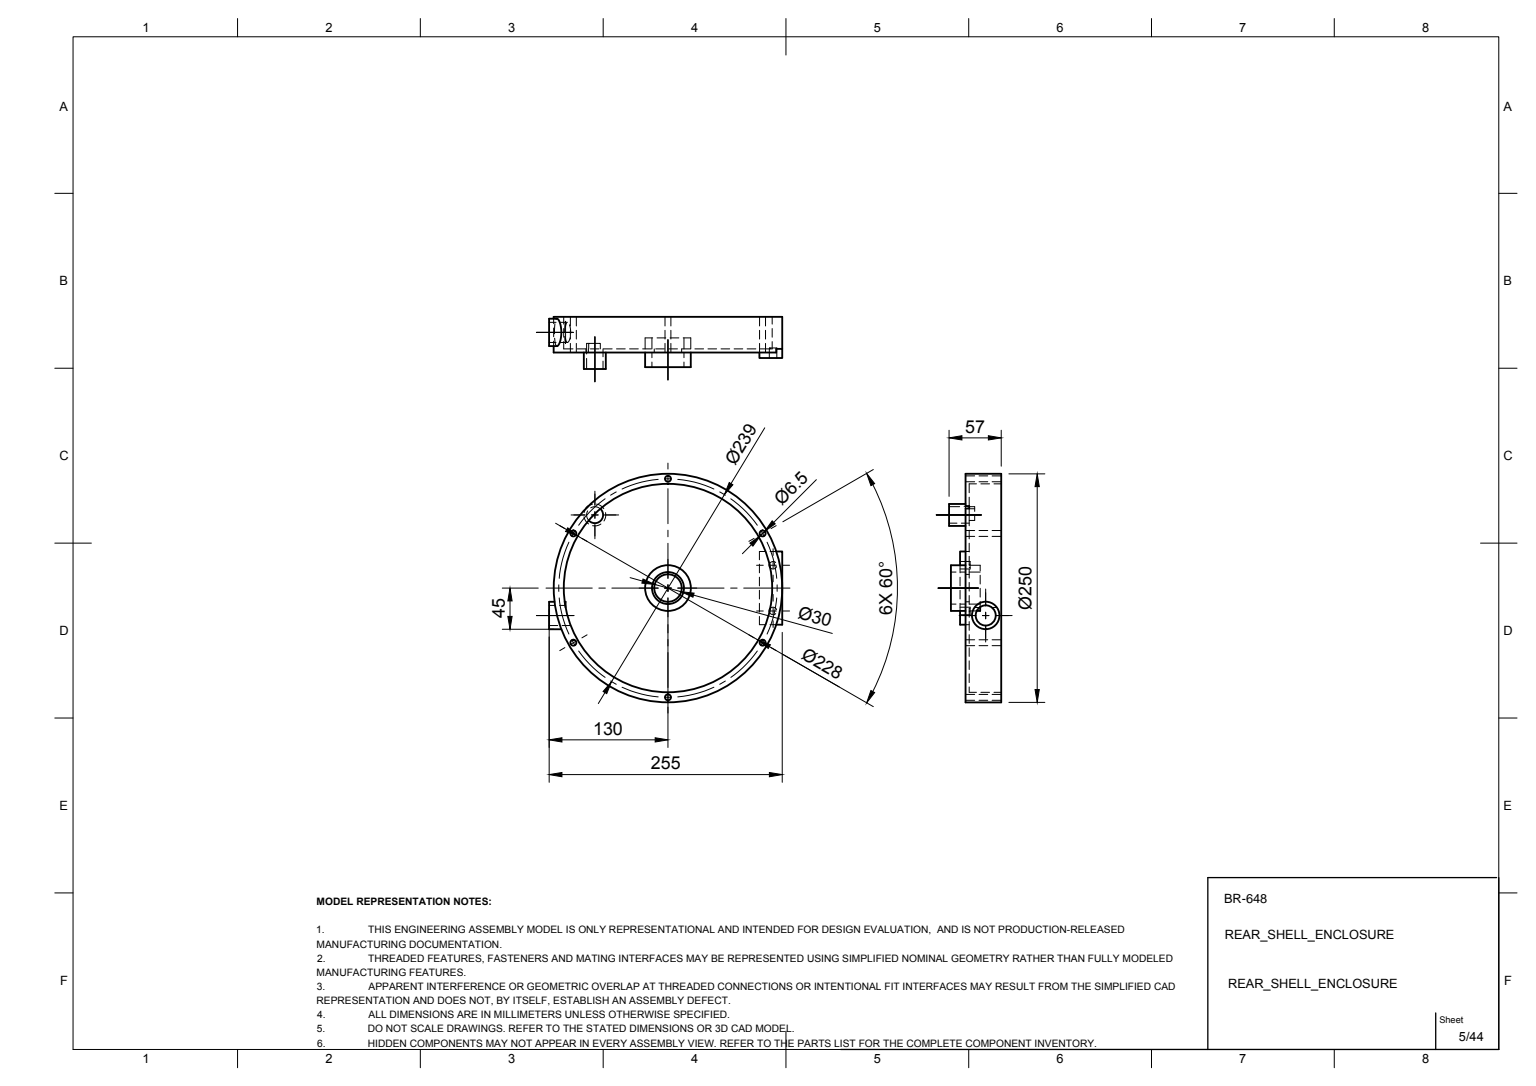
ISO-10303-21;
HEADER;
FILE_DESCRIPTION((''),'2;1');
FILE_NAME('REAR_SHELL_ENCLOSURE.step','2026-10-01T22:05:39-07:00',(''),(''),'','','');
FILE_SCHEMA (('AUTOMOTIVE_DESIGN { 1 0 10303 214 3 1 1 }'));
ENDSEC;
DATA;
#10=MECHANICAL_DESIGN_GEOMETRIC_PRESENTATION_REPRESENTATION('',(#605),#24628);
#521=SHAPE_REPRESENTATION_RELATIONSHIP('SRR','None',#24793,#563) ;
#563=ADVANCED_BREP_SHAPE_REPRESENTATION('',(#647),#24583) ;
#605=STYLED_ITEM('',(#25031),#647) ;
#647=MANIFOLD_SOLID_BREP('REAR_SHELL_ENCLOSURE',#13114) ;
#686=FACE_BOUND('',#3722,.T.) ;
#687=FACE_BOUND('',#3726,.T.) ;
#688=FACE_BOUND('',#3738,.T.) ;
#689=FACE_BOUND('',#3739,.T.) ;
#690=FACE_BOUND('',#3743,.T.) ;
#691=FACE_BOUND('',#3748,.T.) ;
#692=FACE_BOUND('',#3755,.T.) ;
#693=FACE_BOUND('',#3757,.T.) ;
#694=FACE_BOUND('',#3758,.T.) ;
#695=FACE_BOUND('',#3759,.T.) ;
#696=FACE_BOUND('',#3760,.T.) ;
#697=FACE_BOUND('',#3761,.T.) ;
#698=FACE_BOUND('',#3762,.T.) ;
#699=FACE_BOUND('',#3763,.T.) ;
#700=FACE_BOUND('',#3767,.T.) ;
#701=FACE_BOUND('',#3770,.T.) ;
#702=FACE_BOUND('',#3773,.T.) ;
#703=FACE_BOUND('',#3776,.T.) ;
#704=FACE_BOUND('',#3778,.T.) ;
#705=FACE_BOUND('',#3779,.T.) ;
#706=FACE_BOUND('',#3780,.T.) ;
#707=FACE_BOUND('',#3781,.T.) ;
#708=FACE_BOUND('',#3782,.T.) ;
#709=FACE_BOUND('',#3783,.T.) ;
#710=FACE_BOUND('',#3784,.T.) ;
#951=B_SPLINE_CURVE_WITH_KNOTS('',3,(#19746,#19747,#19748,#19749,#19750,
#19751,#19752,#19753,#19754,#19755,#19756,#19757,#19758,#19759,#19760,#19761),
 .UNSPECIFIED.,.F.,.F.,(4,2,2,2,2,2,2,4),(0.687250434098959,0.82687421960189,
1.25301704446935,1.67915986933681,2.11450443098489,2.54984899263297,2.96432241698031,
3.37879584132764),.UNSPECIFIED.) ;
#952=B_SPLINE_CURVE_WITH_KNOTS('',3,(#19763,#19764,#19765,#19766,#19767,
#19768,#19769,#19770,#19771,#19772,#19773,#19774,#19775,#19776,#19777,#19778),
 .UNSPECIFIED.,.F.,.F.,(4,2,2,2,2,2,2,4),(3.37879584132764,3.79326926567498,
4.20774269002231,4.6430872516704,5.07843181331848,5.50457463818594,5.9307174630534,
6.07034124855633),.UNSPECIFIED.) ;
#953=B_SPLINE_CURVE_WITH_KNOTS('',3,(#19782,#19783,#19784,#19785,#19786,
#19787,#19788,#19789,#19790,#19791,#19792,#19793,#19794,#19795,#19796,#19797,
#19798,#19799,#19800,#19801,#19802,#19803,#19804),.UNSPECIFIED.,.F.,.F.,
(4,2,2,2,2,3,2,2,2,2,4),(-1.37470917955979,-1.12781391794867,-0.8458604384615,
-0.563906958974332,-0.281953479487166,0.,0.281953479487167,0.563906958974333,
0.8458604384615,1.12781391794867,1.37470917955955),.UNSPECIFIED.) ;
#954=B_SPLINE_CURVE_WITH_KNOTS('',3,(#19913,#19914,#19915,#19916,#19917,
#19918,#19919,#19920,#19921,#19922,#19923,#19924,#19925,#19926,#19927,#19928,
#19929,#19930,#19931,#19932,#19933,#19934,#19935,#19936,#19937,#19938),
 .UNSPECIFIED.,.F.,.F.,(4,2,2,2,2,2,2,2,2,2,2,2,4),(0.,0.56410198036302,
0.84615297054453,1.12820396072604,1.41660602376442,1.7050080868028,1.99341014984119,
2.28181221287957,2.87260145541368,3.46339069794779,4.02908355018852,4.31192997630889,
4.59477640242925),.UNSPECIFIED.) ;
#955=B_SPLINE_CURVE_WITH_KNOTS('',3,(#19939,#19940,#19941,#19942,#19943,
#19944,#19945,#19946,#19947,#19948,#19949,#19950,#19951,#19952,#19953,#19954,
#19955,#19956,#19957,#19958,#19959,#19960,#19961,#19962,#19963,#19964),
 .UNSPECIFIED.,.F.,.F.,(4,2,2,2,2,2,2,2,2,2,2,2,4),(4.59477640242925,4.87762282854962,
5.16046925466999,5.72616210691072,6.31695134944483,6.90774059197894,7.19614265501732,
7.4845447180557,7.77294678109409,8.06134884413247,8.34339983431398,8.62545082449549,
9.18955280485851),.UNSPECIFIED.) ;
#1001=LINE('',#19715,#1837) ;
#1002=LINE('',#19717,#1838) ;
#1003=LINE('',#19720,#1839) ;
#1004=LINE('',#19725,#1840) ;
#1005=LINE('',#19729,#1841) ;
#1006=LINE('',#19733,#1842) ;
#1007=LINE('',#19738,#1843) ;
#1008=LINE('',#19742,#1844) ;
#1009=LINE('',#19780,#1845) ;
#1010=LINE('',#19805,#1846) ;
#1011=LINE('',#19810,#1847) ;
#1012=LINE('',#19825,#1848) ;
#1013=LINE('',#19831,#1849) ;
#1014=LINE('',#19837,#1850) ;
#1015=LINE('',#19843,#1851) ;
#1016=LINE('',#19849,#1852) ;
#1017=LINE('',#19855,#1853) ;
#1018=LINE('',#19860,#1854) ;
#1019=LINE('',#19862,#1855) ;
#1020=LINE('',#19864,#1856) ;
#1021=LINE('',#19866,#1857) ;
#1022=LINE('',#19868,#1858) ;
#1023=LINE('',#19869,#1859) ;
#1024=LINE('',#19872,#1860) ;
#1025=LINE('',#19874,#1861) ;
#1026=LINE('',#19875,#1862) ;
#1027=LINE('',#19879,#1863) ;
#1028=LINE('',#19883,#1864) ;
#1029=LINE('',#19884,#1865) ;
#1030=LINE('',#19885,#1866) ;
#1031=LINE('',#19887,#1867) ;
#1032=LINE('',#19891,#1868) ;
#1033=LINE('',#19894,#1869) ;
#1034=LINE('',#19895,#1870) ;
#1035=LINE('',#19900,#1871) ;
#1036=LINE('',#19905,#1872) ;
#1037=LINE('',#19909,#1873) ;
#1038=LINE('',#19968,#1874) ;
#1039=LINE('',#19972,#1875) ;
#1040=LINE('',#19983,#1876) ;
#1041=LINE('',#19990,#1877) ;
#1042=LINE('',#20001,#1878) ;
#1043=LINE('',#20007,#1879) ;
#1044=LINE('',#20014,#1880) ;
#1045=LINE('',#20020,#1881) ;
#1046=LINE('',#20024,#1882) ;
#1837=VECTOR('',#15408,0.41) ;
#1838=VECTOR('',#15409,1.) ;
#1839=VECTOR('',#15412,1.) ;
#1840=VECTOR('',#15417,1.) ;
#1841=VECTOR('',#15420,1.) ;
#1842=VECTOR('',#15423,11.4) ;
#1843=VECTOR('',#15428,1.) ;
#1844=VECTOR('',#15431,1.) ;
#1845=VECTOR('',#15434,1.) ;
#1846=VECTOR('',#15435,1.) ;
#1847=VECTOR('',#15440,0.41) ;
#1848=VECTOR('',#15461,0.325) ;
#1849=VECTOR('',#15468,0.325) ;
#1850=VECTOR('',#15475,0.325) ;
#1851=VECTOR('',#15482,0.325) ;
#1852=VECTOR('',#15489,0.325) ;
#1853=VECTOR('',#15496,0.325) ;
#1854=VECTOR('',#15501,1.) ;
#1855=VECTOR('',#15502,1.) ;
#1856=VECTOR('',#15503,1.) ;
#1857=VECTOR('',#15504,1.) ;
#1858=VECTOR('',#15505,1.) ;
#1859=VECTOR('',#15506,1.) ;
#1860=VECTOR('',#15509,1.) ;
#1861=VECTOR('',#15510,1.) ;
#1862=VECTOR('',#15511,1.) ;
#1863=VECTOR('',#15516,1.) ;
#1864=VECTOR('',#15519,1.) ;
#1865=VECTOR('',#15520,1.) ;
#1866=VECTOR('',#15521,1.) ;
#1867=VECTOR('',#15524,1.) ;
#1868=VECTOR('',#15529,1.) ;
#1869=VECTOR('',#15532,1.) ;
#1870=VECTOR('',#15533,1.) ;
#1871=VECTOR('',#15538,12.5) ;
#1872=VECTOR('',#15543,1.) ;
#1873=VECTOR('',#15546,1.) ;
#1874=VECTOR('',#15553,1.1) ;
#1875=VECTOR('',#15558,1.5) ;
#1876=VECTOR('',#15577,0.9) ;
#1877=VECTOR('',#15586,1.2) ;
#1878=VECTOR('',#15601,1.5) ;
#1879=VECTOR('',#15608,1.75) ;
#1880=VECTOR('',#15617,1.75) ;
#1881=VECTOR('',#15626,2.5) ;
#1882=VECTOR('',#15631,2.5) ;
#2673=CYLINDRICAL_SURFACE('',#13659,0.41) ;
#2674=CYLINDRICAL_SURFACE('',#13662,11.4) ;
#2675=CYLINDRICAL_SURFACE('',#13670,0.41) ;
#2676=CYLINDRICAL_SURFACE('',#13680,0.325) ;
#2677=CYLINDRICAL_SURFACE('',#13683,0.325) ;
#2678=CYLINDRICAL_SURFACE('',#13686,0.325) ;
#2679=CYLINDRICAL_SURFACE('',#13689,0.325) ;
#2680=CYLINDRICAL_SURFACE('',#13692,0.325) ;
#2681=CYLINDRICAL_SURFACE('',#13695,0.325) ;
#2682=CYLINDRICAL_SURFACE('',#13707,12.5) ;
#2683=CYLINDRICAL_SURFACE('',#13713,1.1) ;
#2684=CYLINDRICAL_SURFACE('',#13716,1.5) ;
#2685=CYLINDRICAL_SURFACE('',#13718,1.5) ;
#2686=CYLINDRICAL_SURFACE('',#13724,0.9) ;
#2687=CYLINDRICAL_SURFACE('',#13728,1.2) ;
#2688=CYLINDRICAL_SURFACE('',#13735,1.5) ;
#2689=CYLINDRICAL_SURFACE('',#13738,1.75) ;
#2690=CYLINDRICAL_SURFACE('',#13742,1.75) ;
#2691=CYLINDRICAL_SURFACE('',#13746,2.5) ;
#2692=CYLINDRICAL_SURFACE('',#13749,2.5) ;
#2952=FACE_OUTER_BOUND('',#3719,.T.) ;
#2953=FACE_OUTER_BOUND('',#3720,.T.) ;
#2954=FACE_OUTER_BOUND('',#3721,.T.) ;
#2955=FACE_OUTER_BOUND('',#3723,.T.) ;
#2956=FACE_OUTER_BOUND('',#3724,.T.) ;
#2957=FACE_OUTER_BOUND('',#3725,.T.) ;
#2958=FACE_OUTER_BOUND('',#3727,.T.) ;
#2959=FACE_OUTER_BOUND('',#3728,.T.) ;
#2960=FACE_OUTER_BOUND('',#3729,.T.) ;
#2961=FACE_OUTER_BOUND('',#3730,.T.) ;
#2962=FACE_OUTER_BOUND('',#3731,.T.) ;
#2963=FACE_OUTER_BOUND('',#3732,.T.) ;
#2964=FACE_OUTER_BOUND('',#3733,.T.) ;
#2965=FACE_OUTER_BOUND('',#3734,.T.) ;
#2966=FACE_OUTER_BOUND('',#3735,.T.) ;
#2967=FACE_OUTER_BOUND('',#3736,.T.) ;
#2968=FACE_OUTER_BOUND('',#3737,.T.) ;
#2969=FACE_OUTER_BOUND('',#3740,.T.) ;
#2970=FACE_OUTER_BOUND('',#3741,.T.) ;
#2971=FACE_OUTER_BOUND('',#3742,.T.) ;
#2972=FACE_OUTER_BOUND('',#3744,.T.) ;
#2973=FACE_OUTER_BOUND('',#3745,.T.) ;
#2974=FACE_OUTER_BOUND('',#3746,.T.) ;
#2975=FACE_OUTER_BOUND('',#3747,.T.) ;
#2976=FACE_OUTER_BOUND('',#3749,.T.) ;
#2977=FACE_OUTER_BOUND('',#3750,.T.) ;
#2978=FACE_OUTER_BOUND('',#3751,.T.) ;
#2979=FACE_OUTER_BOUND('',#3752,.T.) ;
#2980=FACE_OUTER_BOUND('',#3753,.T.) ;
#2981=FACE_OUTER_BOUND('',#3754,.T.) ;
#2982=FACE_OUTER_BOUND('',#3756,.T.) ;
#2983=FACE_OUTER_BOUND('',#3764,.T.) ;
#2984=FACE_OUTER_BOUND('',#3765,.T.) ;
#2985=FACE_OUTER_BOUND('',#3766,.T.) ;
#2986=FACE_OUTER_BOUND('',#3768,.T.) ;
#2987=FACE_OUTER_BOUND('',#3769,.T.) ;
#2988=FACE_OUTER_BOUND('',#3771,.T.) ;
#2989=FACE_OUTER_BOUND('',#3772,.T.) ;
#2990=FACE_OUTER_BOUND('',#3774,.T.) ;
#2991=FACE_OUTER_BOUND('',#3775,.T.) ;
#2992=FACE_OUTER_BOUND('',#3777,.T.) ;
#3719=EDGE_LOOP('',(#8487,#8488,#8489)) ;
#3720=EDGE_LOOP('',(#8490,#8491,#8492,#8493,#8494,#8495,#8496,#8497)) ;
#3721=EDGE_LOOP('',(#8498,#8499,#8500,#8501,#8502,#8503,#8504,#8505,#8506,
#8507,#8508,#8509,#8510,#8511,#8512,#8513)) ;
#3722=EDGE_LOOP('',(#8514,#8515,#8516,#8517,#8518)) ;
#3723=EDGE_LOOP('',(#8519,#8520,#8521,#8522,#8523,#8524,#8525,#8526)) ;
#3724=EDGE_LOOP('',(#8527,#8528,#8529)) ;
#3725=EDGE_LOOP('',(#8530,#8531,#8532,#8533,#8534,#8535,#8536,#8537)) ;
#3726=EDGE_LOOP('',(#8538)) ;
#3727=EDGE_LOOP('',(#8539,#8540,#8541,#8542)) ;
#3728=EDGE_LOOP('',(#8543,#8544,#8545,#8546)) ;
#3729=EDGE_LOOP('',(#8547,#8548,#8549,#8550)) ;
#3730=EDGE_LOOP('',(#8551,#8552,#8553,#8554)) ;
#3731=EDGE_LOOP('',(#8555,#8556,#8557,#8558)) ;
#3732=EDGE_LOOP('',(#8559,#8560,#8561,#8562)) ;
#3733=EDGE_LOOP('',(#8563,#8564,#8565,#8566,#8567,#8568)) ;
#3734=EDGE_LOOP('',(#8569,#8570,#8571,#8572)) ;
#3735=EDGE_LOOP('',(#8573,#8574,#8575)) ;
#3736=EDGE_LOOP('',(#8576,#8577,#8578,#8579,#8580)) ;
#3737=EDGE_LOOP('',(#8581,#8582,#8583,#8584)) ;
#3738=EDGE_LOOP('',(#8585)) ;
#3739=EDGE_LOOP('',(#8586)) ;
#3740=EDGE_LOOP('',(#8587,#8588,#8589)) ;
#3741=EDGE_LOOP('',(#8590,#8591,#8592,#8593,#8594,#8595)) ;
#3742=EDGE_LOOP('',(#8596,#8597,#8598,#8599,#8600,#8601,#8602,#8603,#8604,
#8605,#8606,#8607,#8608)) ;
#3743=EDGE_LOOP('',(#8609,#8610)) ;
#3744=EDGE_LOOP('',(#8611,#8612,#8613,#8614,#8615,#8616)) ;
#3745=EDGE_LOOP('',(#8617,#8618,#8619,#8620,#8621)) ;
#3746=EDGE_LOOP('',(#8622,#8623)) ;
#3747=EDGE_LOOP('',(#8624)) ;
#3748=EDGE_LOOP('',(#8625)) ;
#3749=EDGE_LOOP('',(#8626,#8627,#8628,#8629)) ;
#3750=EDGE_LOOP('',(#8630,#8631)) ;
#3751=EDGE_LOOP('',(#8632,#8633,#8634,#8635,#8636,#8637,#8638,#8639)) ;
#3752=EDGE_LOOP('',(#8640,#8641)) ;
#3753=EDGE_LOOP('',(#8642,#8643,#8644,#8645,#8646,#8647,#8648,#8649)) ;
#3754=EDGE_LOOP('',(#8650)) ;
#3755=EDGE_LOOP('',(#8651)) ;
#3756=EDGE_LOOP('',(#8652,#8653,#8654,#8655,#8656,#8657,#8658,#8659)) ;
#3757=EDGE_LOOP('',(#8660)) ;
#3758=EDGE_LOOP('',(#8661)) ;
#3759=EDGE_LOOP('',(#8662)) ;
#3760=EDGE_LOOP('',(#8663)) ;
#3761=EDGE_LOOP('',(#8664)) ;
#3762=EDGE_LOOP('',(#8665)) ;
#3763=EDGE_LOOP('',(#8666)) ;
#3764=EDGE_LOOP('',(#8667,#8668,#8669,#8670)) ;
#3765=EDGE_LOOP('',(#8671,#8672,#8673,#8674)) ;
#3766=EDGE_LOOP('',(#8675)) ;
#3767=EDGE_LOOP('',(#8676)) ;
#3768=EDGE_LOOP('',(#8677,#8678,#8679,#8680)) ;
#3769=EDGE_LOOP('',(#8681)) ;
#3770=EDGE_LOOP('',(#8682)) ;
#3771=EDGE_LOOP('',(#8683,#8684,#8685,#8686)) ;
#3772=EDGE_LOOP('',(#8687)) ;
#3773=EDGE_LOOP('',(#8688)) ;
#3774=EDGE_LOOP('',(#8689,#8690,#8691,#8692)) ;
#3775=EDGE_LOOP('',(#8693)) ;
#3776=EDGE_LOOP('',(#8694)) ;
#3777=EDGE_LOOP('',(#8695)) ;
#3778=EDGE_LOOP('',(#8696)) ;
#3779=EDGE_LOOP('',(#8697)) ;
#3780=EDGE_LOOP('',(#8698)) ;
#3781=EDGE_LOOP('',(#8699)) ;
#3782=EDGE_LOOP('',(#8700)) ;
#3783=EDGE_LOOP('',(#8701)) ;
#3784=EDGE_LOOP('',(#8702)) ;
#4751=CIRCLE('',#13656,11.4) ;
#4752=CIRCLE('',#13657,0.41) ;
#4753=CIRCLE('',#13658,0.41) ;
#4754=CIRCLE('',#13660,0.41) ;
#4755=CIRCLE('',#13661,0.41) ;
#4756=CIRCLE('',#13663,11.4) ;
#4757=CIRCLE('',#13664,11.4) ;
#4758=CIRCLE('',#13665,11.4) ;
#4759=CIRCLE('',#13666,11.4) ;
#4760=CIRCLE('',#13667,11.4) ;
#4761=CIRCLE('',#13668,11.4) ;
#4762=CIRCLE('',#13669,11.4) ;
#4763=CIRCLE('',#13671,0.41) ;
#4764=CIRCLE('',#13672,0.41) ;
#4765=CIRCLE('',#13673,0.41) ;
#4766=CIRCLE('',#13674,0.41) ;
#4767=CIRCLE('',#13677,0.9) ;
#4768=CIRCLE('',#13678,0.9) ;
#4769=CIRCLE('',#13679,2.5) ;
#4770=CIRCLE('',#13681,0.325) ;
#4771=CIRCLE('',#13682,0.325) ;
#4772=CIRCLE('',#13684,0.325) ;
#4773=CIRCLE('',#13685,0.325) ;
#4774=CIRCLE('',#13687,0.325) ;
#4775=CIRCLE('',#13688,0.325) ;
#4776=CIRCLE('',#13690,0.325) ;
#4777=CIRCLE('',#13691,0.325) ;
#4778=CIRCLE('',#13693,0.325) ;
#4779=CIRCLE('',#13694,0.325) ;
#4780=CIRCLE('',#13696,0.325) ;
#4781=CIRCLE('',#13697,0.325) ;
#4782=CIRCLE('',#13701,12.5) ;
#4783=CIRCLE('',#13705,12.5) ;
#4784=CIRCLE('',#13708,12.5) ;
#4785=CIRCLE('',#13709,12.5) ;
#4786=CIRCLE('',#13710,12.5) ;
#4787=CIRCLE('',#13711,12.5) ;
#4788=CIRCLE('',#13712,12.5) ;
#4789=CIRCLE('',#13714,1.1) ;
#4790=CIRCLE('',#13715,1.1) ;
#4791=CIRCLE('',#13717,1.5) ;
#4792=CIRCLE('',#13719,1.5) ;
#4793=CIRCLE('',#13723,0.9) ;
#4794=CIRCLE('',#13725,0.9) ;
#4795=CIRCLE('',#13727,1.2) ;
#4796=CIRCLE('',#13729,1.2) ;
#4797=CIRCLE('',#13730,1.2) ;
#4798=CIRCLE('',#13731,1.2) ;
#4799=CIRCLE('',#13734,2.5) ;
#4800=CIRCLE('',#13736,1.5) ;
#4801=CIRCLE('',#13737,1.5) ;
#4802=CIRCLE('',#13739,1.75) ;
#4803=CIRCLE('',#13740,1.75) ;
#4804=CIRCLE('',#13743,1.75) ;
#4805=CIRCLE('',#13744,1.75) ;
#4806=CIRCLE('',#13747,2.5) ;
#4807=CIRCLE('',#13750,2.5) ;
#5537=VERTEX_POINT('',#19706) ;
#5538=VERTEX_POINT('',#19707) ;
#5539=VERTEX_POINT('',#19709) ;
#5540=VERTEX_POINT('',#19713) ;
#5541=VERTEX_POINT('',#19716) ;
#5542=VERTEX_POINT('',#19718) ;
#5543=VERTEX_POINT('',#19722) ;
#5544=VERTEX_POINT('',#19724) ;
#5545=VERTEX_POINT('',#19726) ;
#5546=VERTEX_POINT('',#19728) ;
#5547=VERTEX_POINT('',#19730) ;
#5548=VERTEX_POINT('',#19732) ;
#5549=VERTEX_POINT('',#19735) ;
#5550=VERTEX_POINT('',#19737) ;
#5551=VERTEX_POINT('',#19739) ;
#5552=VERTEX_POINT('',#19741) ;
#5553=VERTEX_POINT('',#19744) ;
#5554=VERTEX_POINT('',#19745) ;
#5555=VERTEX_POINT('',#19762) ;
#5556=VERTEX_POINT('',#19779) ;
#5557=VERTEX_POINT('',#19781) ;
#5558=VERTEX_POINT('',#19807) ;
#5559=VERTEX_POINT('',#19809) ;
#5560=VERTEX_POINT('',#19816) ;
#5561=VERTEX_POINT('',#19819) ;
#5562=VERTEX_POINT('',#19822) ;
#5563=VERTEX_POINT('',#19824) ;
#5564=VERTEX_POINT('',#19828) ;
#5565=VERTEX_POINT('',#19830) ;
#5566=VERTEX_POINT('',#19834) ;
#5567=VERTEX_POINT('',#19836) ;
#5568=VERTEX_POINT('',#19840) ;
#5569=VERTEX_POINT('',#19842) ;
#5570=VERTEX_POINT('',#19846) ;
#5571=VERTEX_POINT('',#19848) ;
#5572=VERTEX_POINT('',#19852) ;
#5573=VERTEX_POINT('',#19854) ;
#5574=VERTEX_POINT('',#19858) ;
#5575=VERTEX_POINT('',#19859) ;
#5576=VERTEX_POINT('',#19861) ;
#5577=VERTEX_POINT('',#19863) ;
#5578=VERTEX_POINT('',#19865) ;
#5579=VERTEX_POINT('',#19867) ;
#5580=VERTEX_POINT('',#19871) ;
#5581=VERTEX_POINT('',#19873) ;
#5582=VERTEX_POINT('',#19877) ;
#5583=VERTEX_POINT('',#19881) ;
#5584=VERTEX_POINT('',#19882) ;
#5585=VERTEX_POINT('',#19889) ;
#5586=VERTEX_POINT('',#19893) ;
#5587=VERTEX_POINT('',#19897) ;
#5588=VERTEX_POINT('',#19899) ;
#5589=VERTEX_POINT('',#19902) ;
#5590=VERTEX_POINT('',#19904) ;
#5591=VERTEX_POINT('',#19906) ;
#5592=VERTEX_POINT('',#19908) ;
#5593=VERTEX_POINT('',#19911) ;
#5594=VERTEX_POINT('',#19912) ;
#5595=VERTEX_POINT('',#19966) ;
#5596=VERTEX_POINT('',#19971) ;
#5597=VERTEX_POINT('',#19981) ;
#5598=VERTEX_POINT('',#19987) ;
#5599=VERTEX_POINT('',#19989) ;
#5600=VERTEX_POINT('',#19995) ;
#5601=VERTEX_POINT('',#19998) ;
#5602=VERTEX_POINT('',#20000) ;
#5603=VERTEX_POINT('',#20004) ;
#5604=VERTEX_POINT('',#20006) ;
#5605=VERTEX_POINT('',#20011) ;
#5606=VERTEX_POINT('',#20013) ;
#5607=VERTEX_POINT('',#20018) ;
#5608=VERTEX_POINT('',#20023) ;
#6733=EDGE_CURVE('',#5537,#5538,#4751,.T.) ;
#6734=EDGE_CURVE('',#5539,#5537,#4752,.T.) ;
#6735=EDGE_CURVE('',#5538,#5539,#4753,.T.) ;
#6736=EDGE_CURVE('',#5540,#5540,#4754,.T.) ;
#6737=EDGE_CURVE('',#5540,#5539,#1001,.T.) ;
#6738=EDGE_CURVE('',#5541,#5537,#1002,.T.) ;
#6739=EDGE_CURVE('',#5542,#5541,#4755,.T.) ;
#6740=EDGE_CURVE('',#5538,#5542,#1003,.T.) ;
#6741=EDGE_CURVE('',#5542,#5543,#4756,.T.) ;
#6742=EDGE_CURVE('',#5543,#5544,#1004,.T.) ;
#6743=EDGE_CURVE('',#5544,#5545,#4757,.T.) ;
#6744=EDGE_CURVE('',#5545,#5546,#1005,.T.) ;
#6745=EDGE_CURVE('',#5546,#5547,#4758,.T.) ;
#6746=EDGE_CURVE('',#5547,#5548,#1006,.T.) ;
#6747=EDGE_CURVE('',#5548,#5548,#4759,.T.) ;
#6748=EDGE_CURVE('',#5547,#5549,#4760,.T.) ;
#6749=EDGE_CURVE('',#5549,#5550,#1007,.T.) ;
#6750=EDGE_CURVE('',#5550,#5551,#4761,.T.) ;
#6751=EDGE_CURVE('',#5551,#5552,#1008,.T.) ;
#6752=EDGE_CURVE('',#5552,#5541,#4762,.T.) ;
#6753=EDGE_CURVE('',#5553,#5554,#951,.T.) ;
#6754=EDGE_CURVE('',#5554,#5555,#952,.T.) ;
#6755=EDGE_CURVE('',#5555,#5556,#1009,.T.) ;
#6756=EDGE_CURVE('',#5556,#5557,#953,.T.) ;
#6757=EDGE_CURVE('',#5557,#5553,#1010,.T.) ;
#6758=EDGE_CURVE('',#5558,#5558,#4763,.T.) ;
#6759=EDGE_CURVE('',#5558,#5559,#1011,.T.) ;
#6760=EDGE_CURVE('',#5559,#5544,#4764,.T.) ;
#6761=EDGE_CURVE('',#5546,#5543,#4765,.T.) ;
#6762=EDGE_CURVE('',#5545,#5559,#4766,.T.) ;
#6763=EDGE_CURVE('',#5552,#5560,#4767,.T.) ;
#6764=EDGE_CURVE('',#5560,#5549,#4768,.T.) ;
#6765=EDGE_CURVE('',#5561,#5561,#4769,.T.) ;
#6766=EDGE_CURVE('',#5562,#5562,#4770,.T.) ;
#6767=EDGE_CURVE('',#5562,#5563,#1012,.T.) ;
#6768=EDGE_CURVE('',#5563,#5563,#4771,.T.) ;
#6769=EDGE_CURVE('',#5564,#5564,#4772,.T.) ;
#6770=EDGE_CURVE('',#5564,#5565,#1013,.T.) ;
#6771=EDGE_CURVE('',#5565,#5565,#4773,.T.) ;
#6772=EDGE_CURVE('',#5566,#5566,#4774,.T.) ;
#6773=EDGE_CURVE('',#5566,#5567,#1014,.T.) ;
#6774=EDGE_CURVE('',#5567,#5567,#4775,.T.) ;
#6775=EDGE_CURVE('',#5568,#5568,#4776,.T.) ;
#6776=EDGE_CURVE('',#5568,#5569,#1015,.T.) ;
#6777=EDGE_CURVE('',#5569,#5569,#4777,.T.) ;
#6778=EDGE_CURVE('',#5570,#5570,#4778,.T.) ;
#6779=EDGE_CURVE('',#5570,#5571,#1016,.T.) ;
#6780=EDGE_CURVE('',#5571,#5571,#4779,.T.) ;
#6781=EDGE_CURVE('',#5572,#5572,#4780,.T.) ;
#6782=EDGE_CURVE('',#5572,#5573,#1017,.T.) ;
#6783=EDGE_CURVE('',#5573,#5573,#4781,.T.) ;
#6784=EDGE_CURVE('',#5574,#5575,#1018,.T.) ;
#6785=EDGE_CURVE('',#5576,#5574,#1019,.T.) ;
#6786=EDGE_CURVE('',#5577,#5576,#1020,.T.) ;
#6787=EDGE_CURVE('',#5578,#5577,#1021,.T.) ;
#6788=EDGE_CURVE('',#5579,#5578,#1022,.T.) ;
#6789=EDGE_CURVE('',#5579,#5575,#1023,.T.) ;
#6790=EDGE_CURVE('',#5580,#5576,#1024,.T.) ;
#6791=EDGE_CURVE('',#5580,#5581,#1025,.T.) ;
#6792=EDGE_CURVE('',#5581,#5577,#1026,.T.) ;
#6793=EDGE_CURVE('',#5575,#5582,#4782,.T.) ;
#6794=EDGE_CURVE('',#5582,#5579,#1027,.T.) ;
#6795=EDGE_CURVE('',#5583,#5584,#1028,.T.) ;
#6796=EDGE_CURVE('',#5584,#5582,#1029,.T.) ;
#6797=EDGE_CURVE('',#5578,#5583,#1030,.T.) ;
#6798=EDGE_CURVE('',#5583,#5581,#1031,.T.) ;
#6799=EDGE_CURVE('',#5582,#5585,#4783,.T.) ;
#6800=EDGE_CURVE('',#5584,#5585,#1032,.T.) ;
#6801=EDGE_CURVE('',#5585,#5586,#1033,.T.) ;
#6802=EDGE_CURVE('',#5586,#5580,#1034,.T.) ;
#6803=EDGE_CURVE('',#5587,#5587,#4784,.T.) ;
#6804=EDGE_CURVE('',#5587,#5588,#1035,.T.) ;
#6805=EDGE_CURVE('',#5574,#5588,#4785,.T.) ;
#6806=EDGE_CURVE('',#5589,#5586,#4786,.T.) ;
#6807=EDGE_CURVE('',#5589,#5590,#1036,.T.) ;
#6808=EDGE_CURVE('',#5590,#5591,#4787,.T.) ;
#6809=EDGE_CURVE('',#5591,#5592,#1037,.T.) ;
#6810=EDGE_CURVE('',#5588,#5592,#4788,.T.) ;
#6811=EDGE_CURVE('',#5593,#5594,#954,.T.) ;
#6812=EDGE_CURVE('',#5594,#5593,#955,.T.) ;
#6813=EDGE_CURVE('',#5595,#5595,#4789,.T.) ;
#6814=EDGE_CURVE('',#5595,#5554,#1038,.T.) ;
#6815=EDGE_CURVE('',#5555,#5553,#4790,.T.) ;
#6816=EDGE_CURVE('',#5594,#5596,#1039,.T.) ;
#6817=EDGE_CURVE('',#5596,#5596,#4791,.T.) ;
#6818=EDGE_CURVE('',#5557,#5556,#4792,.T.) ;
#6819=EDGE_CURVE('',#5551,#5550,#4793,.T.) ;
#6820=EDGE_CURVE('',#5597,#5597,#4794,.T.) ;
#6821=EDGE_CURVE('',#5597,#5560,#1040,.T.) ;
#6822=EDGE_CURVE('',#5590,#5591,#4795,.T.) ;
#6823=EDGE_CURVE('',#5598,#5589,#4796,.T.) ;
#6824=EDGE_CURVE('',#5598,#5599,#1041,.T.) ;
#6825=EDGE_CURVE('',#5599,#5599,#4797,.T.) ;
#6826=EDGE_CURVE('',#5592,#5598,#4798,.T.) ;
#6827=EDGE_CURVE('',#5600,#5600,#4799,.T.) ;
#6828=EDGE_CURVE('',#5601,#5601,#4800,.T.) ;
#6829=EDGE_CURVE('',#5601,#5602,#1042,.T.) ;
#6830=EDGE_CURVE('',#5602,#5602,#4801,.T.) ;
#6831=EDGE_CURVE('',#5603,#5603,#4802,.T.) ;
#6832=EDGE_CURVE('',#5603,#5604,#1043,.T.) ;
#6833=EDGE_CURVE('',#5604,#5604,#4803,.T.) ;
#6834=EDGE_CURVE('',#5605,#5605,#4804,.T.) ;
#6835=EDGE_CURVE('',#5605,#5606,#1044,.T.) ;
#6836=EDGE_CURVE('',#5606,#5606,#4805,.T.) ;
#6837=EDGE_CURVE('',#5607,#5607,#4806,.T.) ;
#6838=EDGE_CURVE('',#5607,#5561,#1045,.T.) ;
#6839=EDGE_CURVE('',#5600,#5608,#1046,.T.) ;
#6840=EDGE_CURVE('',#5608,#5608,#4807,.T.) ;
#8487=ORIENTED_EDGE('',*,*,#6733,.F.) ;
#8488=ORIENTED_EDGE('',*,*,#6734,.F.) ;
#8489=ORIENTED_EDGE('',*,*,#6735,.F.) ;
#8490=ORIENTED_EDGE('',*,*,#6736,.F.) ;
#8491=ORIENTED_EDGE('',*,*,#6737,.T.) ;
#8492=ORIENTED_EDGE('',*,*,#6734,.T.) ;
#8493=ORIENTED_EDGE('',*,*,#6738,.F.) ;
#8494=ORIENTED_EDGE('',*,*,#6739,.F.) ;
#8495=ORIENTED_EDGE('',*,*,#6740,.F.) ;
#8496=ORIENTED_EDGE('',*,*,#6735,.T.) ;
#8497=ORIENTED_EDGE('',*,*,#6737,.F.) ;
#8498=ORIENTED_EDGE('',*,*,#6738,.T.) ;
#8499=ORIENTED_EDGE('',*,*,#6733,.T.) ;
#8500=ORIENTED_EDGE('',*,*,#6740,.T.) ;
#8501=ORIENTED_EDGE('',*,*,#6741,.T.) ;
#8502=ORIENTED_EDGE('',*,*,#6742,.T.) ;
#8503=ORIENTED_EDGE('',*,*,#6743,.T.) ;
#8504=ORIENTED_EDGE('',*,*,#6744,.T.) ;
#8505=ORIENTED_EDGE('',*,*,#6745,.T.) ;
#8506=ORIENTED_EDGE('',*,*,#6746,.T.) ;
#8507=ORIENTED_EDGE('',*,*,#6747,.F.) ;
#8508=ORIENTED_EDGE('',*,*,#6746,.F.) ;
#8509=ORIENTED_EDGE('',*,*,#6748,.T.) ;
#8510=ORIENTED_EDGE('',*,*,#6749,.T.) ;
#8511=ORIENTED_EDGE('',*,*,#6750,.T.) ;
#8512=ORIENTED_EDGE('',*,*,#6751,.T.) ;
#8513=ORIENTED_EDGE('',*,*,#6752,.T.) ;
#8514=ORIENTED_EDGE('',*,*,#6753,.T.) ;
#8515=ORIENTED_EDGE('',*,*,#6754,.T.) ;
#8516=ORIENTED_EDGE('',*,*,#6755,.T.) ;
#8517=ORIENTED_EDGE('',*,*,#6756,.T.) ;
#8518=ORIENTED_EDGE('',*,*,#6757,.T.) ;
#8519=ORIENTED_EDGE('',*,*,#6758,.F.) ;
#8520=ORIENTED_EDGE('',*,*,#6759,.T.) ;
#8521=ORIENTED_EDGE('',*,*,#6760,.T.) ;
#8522=ORIENTED_EDGE('',*,*,#6742,.F.) ;
#8523=ORIENTED_EDGE('',*,*,#6761,.F.) ;
#8524=ORIENTED_EDGE('',*,*,#6744,.F.) ;
#8525=ORIENTED_EDGE('',*,*,#6762,.T.) ;
#8526=ORIENTED_EDGE('',*,*,#6759,.F.) ;
#8527=ORIENTED_EDGE('',*,*,#6743,.F.) ;
#8528=ORIENTED_EDGE('',*,*,#6760,.F.) ;
#8529=ORIENTED_EDGE('',*,*,#6762,.F.) ;
#8530=ORIENTED_EDGE('',*,*,#6739,.T.) ;
#8531=ORIENTED_EDGE('',*,*,#6752,.F.) ;
#8532=ORIENTED_EDGE('',*,*,#6763,.T.) ;
#8533=ORIENTED_EDGE('',*,*,#6764,.T.) ;
#8534=ORIENTED_EDGE('',*,*,#6748,.F.) ;
#8535=ORIENTED_EDGE('',*,*,#6745,.F.) ;
#8536=ORIENTED_EDGE('',*,*,#6761,.T.) ;
#8537=ORIENTED_EDGE('',*,*,#6741,.F.) ;
#8538=ORIENTED_EDGE('',*,*,#6765,.T.) ;
#8539=ORIENTED_EDGE('',*,*,#6766,.F.) ;
#8540=ORIENTED_EDGE('',*,*,#6767,.T.) ;
#8541=ORIENTED_EDGE('',*,*,#6768,.F.) ;
#8542=ORIENTED_EDGE('',*,*,#6767,.F.) ;
#8543=ORIENTED_EDGE('',*,*,#6769,.F.) ;
#8544=ORIENTED_EDGE('',*,*,#6770,.T.) ;
#8545=ORIENTED_EDGE('',*,*,#6771,.F.) ;
#8546=ORIENTED_EDGE('',*,*,#6770,.F.) ;
#8547=ORIENTED_EDGE('',*,*,#6772,.F.) ;
#8548=ORIENTED_EDGE('',*,*,#6773,.T.) ;
#8549=ORIENTED_EDGE('',*,*,#6774,.F.) ;
#8550=ORIENTED_EDGE('',*,*,#6773,.F.) ;
#8551=ORIENTED_EDGE('',*,*,#6775,.F.) ;
#8552=ORIENTED_EDGE('',*,*,#6776,.T.) ;
#8553=ORIENTED_EDGE('',*,*,#6777,.F.) ;
#8554=ORIENTED_EDGE('',*,*,#6776,.F.) ;
#8555=ORIENTED_EDGE('',*,*,#6778,.F.) ;
#8556=ORIENTED_EDGE('',*,*,#6779,.T.) ;
#8557=ORIENTED_EDGE('',*,*,#6780,.F.) ;
#8558=ORIENTED_EDGE('',*,*,#6779,.F.) ;
#8559=ORIENTED_EDGE('',*,*,#6781,.F.) ;
#8560=ORIENTED_EDGE('',*,*,#6782,.T.) ;
#8561=ORIENTED_EDGE('',*,*,#6783,.F.) ;
#8562=ORIENTED_EDGE('',*,*,#6782,.F.) ;
#8563=ORIENTED_EDGE('',*,*,#6784,.F.) ;
#8564=ORIENTED_EDGE('',*,*,#6785,.F.) ;
#8565=ORIENTED_EDGE('',*,*,#6786,.F.) ;
#8566=ORIENTED_EDGE('',*,*,#6787,.F.) ;
#8567=ORIENTED_EDGE('',*,*,#6788,.F.) ;
#8568=ORIENTED_EDGE('',*,*,#6789,.T.) ;
#8569=ORIENTED_EDGE('',*,*,#6790,.F.) ;
#8570=ORIENTED_EDGE('',*,*,#6791,.T.) ;
#8571=ORIENTED_EDGE('',*,*,#6792,.T.) ;
#8572=ORIENTED_EDGE('',*,*,#6786,.T.) ;
#8573=ORIENTED_EDGE('',*,*,#6793,.F.) ;
#8574=ORIENTED_EDGE('',*,*,#6789,.F.) ;
#8575=ORIENTED_EDGE('',*,*,#6794,.F.) ;
#8576=ORIENTED_EDGE('',*,*,#6795,.T.) ;
#8577=ORIENTED_EDGE('',*,*,#6796,.T.) ;
#8578=ORIENTED_EDGE('',*,*,#6794,.T.) ;
#8579=ORIENTED_EDGE('',*,*,#6788,.T.) ;
#8580=ORIENTED_EDGE('',*,*,#6797,.T.) ;
#8581=ORIENTED_EDGE('',*,*,#6787,.T.) ;
#8582=ORIENTED_EDGE('',*,*,#6792,.F.) ;
#8583=ORIENTED_EDGE('',*,*,#6798,.F.) ;
#8584=ORIENTED_EDGE('',*,*,#6797,.F.) ;
#8585=ORIENTED_EDGE('',*,*,#6736,.T.) ;
#8586=ORIENTED_EDGE('',*,*,#6758,.T.) ;
#8587=ORIENTED_EDGE('',*,*,#6799,.F.) ;
#8588=ORIENTED_EDGE('',*,*,#6796,.F.) ;
#8589=ORIENTED_EDGE('',*,*,#6800,.T.) ;
#8590=ORIENTED_EDGE('',*,*,#6801,.F.) ;
#8591=ORIENTED_EDGE('',*,*,#6800,.F.) ;
#8592=ORIENTED_EDGE('',*,*,#6795,.F.) ;
#8593=ORIENTED_EDGE('',*,*,#6798,.T.) ;
#8594=ORIENTED_EDGE('',*,*,#6791,.F.) ;
#8595=ORIENTED_EDGE('',*,*,#6802,.F.) ;
#8596=ORIENTED_EDGE('',*,*,#6803,.F.) ;
#8597=ORIENTED_EDGE('',*,*,#6804,.T.) ;
#8598=ORIENTED_EDGE('',*,*,#6805,.F.) ;
#8599=ORIENTED_EDGE('',*,*,#6784,.T.) ;
#8600=ORIENTED_EDGE('',*,*,#6793,.T.) ;
#8601=ORIENTED_EDGE('',*,*,#6799,.T.) ;
#8602=ORIENTED_EDGE('',*,*,#6801,.T.) ;
#8603=ORIENTED_EDGE('',*,*,#6806,.F.) ;
#8604=ORIENTED_EDGE('',*,*,#6807,.T.) ;
#8605=ORIENTED_EDGE('',*,*,#6808,.T.) ;
#8606=ORIENTED_EDGE('',*,*,#6809,.T.) ;
#8607=ORIENTED_EDGE('',*,*,#6810,.F.) ;
#8608=ORIENTED_EDGE('',*,*,#6804,.F.) ;
#8609=ORIENTED_EDGE('',*,*,#6811,.T.) ;
#8610=ORIENTED_EDGE('',*,*,#6812,.T.) ;
#8611=ORIENTED_EDGE('',*,*,#6813,.F.) ;
#8612=ORIENTED_EDGE('',*,*,#6814,.T.) ;
#8613=ORIENTED_EDGE('',*,*,#6753,.F.) ;
#8614=ORIENTED_EDGE('',*,*,#6815,.F.) ;
#8615=ORIENTED_EDGE('',*,*,#6754,.F.) ;
#8616=ORIENTED_EDGE('',*,*,#6814,.F.) ;
#8617=ORIENTED_EDGE('',*,*,#6811,.F.) ;
#8618=ORIENTED_EDGE('',*,*,#6812,.F.) ;
#8619=ORIENTED_EDGE('',*,*,#6816,.T.) ;
#8620=ORIENTED_EDGE('',*,*,#6817,.F.) ;
#8621=ORIENTED_EDGE('',*,*,#6816,.F.) ;
#8622=ORIENTED_EDGE('',*,*,#6756,.F.) ;
#8623=ORIENTED_EDGE('',*,*,#6818,.F.) ;
#8624=ORIENTED_EDGE('',*,*,#6817,.T.) ;
#8625=ORIENTED_EDGE('',*,*,#6813,.T.) ;
#8626=ORIENTED_EDGE('',*,*,#6815,.T.) ;
#8627=ORIENTED_EDGE('',*,*,#6757,.F.) ;
#8628=ORIENTED_EDGE('',*,*,#6818,.T.) ;
#8629=ORIENTED_EDGE('',*,*,#6755,.F.) ;
#8630=ORIENTED_EDGE('',*,*,#6750,.F.) ;
#8631=ORIENTED_EDGE('',*,*,#6819,.F.) ;
#8632=ORIENTED_EDGE('',*,*,#6820,.F.) ;
#8633=ORIENTED_EDGE('',*,*,#6821,.T.) ;
#8634=ORIENTED_EDGE('',*,*,#6763,.F.) ;
#8635=ORIENTED_EDGE('',*,*,#6751,.F.) ;
#8636=ORIENTED_EDGE('',*,*,#6819,.T.) ;
#8637=ORIENTED_EDGE('',*,*,#6749,.F.) ;
#8638=ORIENTED_EDGE('',*,*,#6764,.F.) ;
#8639=ORIENTED_EDGE('',*,*,#6821,.F.) ;
#8640=ORIENTED_EDGE('',*,*,#6808,.F.) ;
#8641=ORIENTED_EDGE('',*,*,#6822,.T.) ;
#8642=ORIENTED_EDGE('',*,*,#6809,.F.) ;
#8643=ORIENTED_EDGE('',*,*,#6822,.F.) ;
#8644=ORIENTED_EDGE('',*,*,#6807,.F.) ;
#8645=ORIENTED_EDGE('',*,*,#6823,.F.) ;
#8646=ORIENTED_EDGE('',*,*,#6824,.T.) ;
#8647=ORIENTED_EDGE('',*,*,#6825,.F.) ;
#8648=ORIENTED_EDGE('',*,*,#6824,.F.) ;
#8649=ORIENTED_EDGE('',*,*,#6826,.F.) ;
#8650=ORIENTED_EDGE('',*,*,#6825,.T.) ;
#8651=ORIENTED_EDGE('',*,*,#6820,.T.) ;
#8652=ORIENTED_EDGE('',*,*,#6785,.T.) ;
#8653=ORIENTED_EDGE('',*,*,#6805,.T.) ;
#8654=ORIENTED_EDGE('',*,*,#6810,.T.) ;
#8655=ORIENTED_EDGE('',*,*,#6826,.T.) ;
#8656=ORIENTED_EDGE('',*,*,#6823,.T.) ;
#8657=ORIENTED_EDGE('',*,*,#6806,.T.) ;
#8658=ORIENTED_EDGE('',*,*,#6802,.T.) ;
#8659=ORIENTED_EDGE('',*,*,#6790,.T.) ;
#8660=ORIENTED_EDGE('',*,*,#6766,.T.) ;
#8661=ORIENTED_EDGE('',*,*,#6769,.T.) ;
#8662=ORIENTED_EDGE('',*,*,#6772,.T.) ;
#8663=ORIENTED_EDGE('',*,*,#6775,.T.) ;
#8664=ORIENTED_EDGE('',*,*,#6778,.T.) ;
#8665=ORIENTED_EDGE('',*,*,#6781,.T.) ;
#8666=ORIENTED_EDGE('',*,*,#6827,.T.) ;
#8667=ORIENTED_EDGE('',*,*,#6828,.F.) ;
#8668=ORIENTED_EDGE('',*,*,#6829,.T.) ;
#8669=ORIENTED_EDGE('',*,*,#6830,.F.) ;
#8670=ORIENTED_EDGE('',*,*,#6829,.F.) ;
#8671=ORIENTED_EDGE('',*,*,#6831,.T.) ;
#8672=ORIENTED_EDGE('',*,*,#6832,.T.) ;
#8673=ORIENTED_EDGE('',*,*,#6833,.F.) ;
#8674=ORIENTED_EDGE('',*,*,#6832,.F.) ;
#8675=ORIENTED_EDGE('',*,*,#6831,.F.) ;
#8676=ORIENTED_EDGE('',*,*,#6830,.T.) ;
#8677=ORIENTED_EDGE('',*,*,#6834,.F.) ;
#8678=ORIENTED_EDGE('',*,*,#6835,.T.) ;
#8679=ORIENTED_EDGE('',*,*,#6836,.T.) ;
#8680=ORIENTED_EDGE('',*,*,#6835,.F.) ;
#8681=ORIENTED_EDGE('',*,*,#6836,.F.) ;
#8682=ORIENTED_EDGE('',*,*,#6828,.T.) ;
#8683=ORIENTED_EDGE('',*,*,#6837,.F.) ;
#8684=ORIENTED_EDGE('',*,*,#6838,.T.) ;
#8685=ORIENTED_EDGE('',*,*,#6765,.F.) ;
#8686=ORIENTED_EDGE('',*,*,#6838,.F.) ;
#8687=ORIENTED_EDGE('',*,*,#6837,.T.) ;
#8688=ORIENTED_EDGE('',*,*,#6833,.T.) ;
#8689=ORIENTED_EDGE('',*,*,#6827,.F.) ;
#8690=ORIENTED_EDGE('',*,*,#6839,.T.) ;
#8691=ORIENTED_EDGE('',*,*,#6840,.F.) ;
#8692=ORIENTED_EDGE('',*,*,#6839,.F.) ;
#8693=ORIENTED_EDGE('',*,*,#6840,.T.) ;
#8694=ORIENTED_EDGE('',*,*,#6834,.T.) ;
#8695=ORIENTED_EDGE('',*,*,#6803,.T.) ;
#8696=ORIENTED_EDGE('',*,*,#6768,.T.) ;
#8697=ORIENTED_EDGE('',*,*,#6771,.T.) ;
#8698=ORIENTED_EDGE('',*,*,#6774,.T.) ;
#8699=ORIENTED_EDGE('',*,*,#6777,.T.) ;
#8700=ORIENTED_EDGE('',*,*,#6780,.T.) ;
#8701=ORIENTED_EDGE('',*,*,#6783,.T.) ;
#8702=ORIENTED_EDGE('',*,*,#6747,.T.) ;
#11995=PLANE('',#13655) ;
#11996=PLANE('',#13675) ;
#11997=PLANE('',#13676) ;
#11998=PLANE('',#13698) ;
#11999=PLANE('',#13699) ;
#12000=PLANE('',#13700) ;
#12001=PLANE('',#13702) ;
#12002=PLANE('',#13703) ;
#12003=PLANE('',#13704) ;
#12004=PLANE('',#13706) ;
#12005=PLANE('',#13720) ;
#12006=PLANE('',#13721) ;
#12007=PLANE('',#13722) ;
#12008=PLANE('',#13726) ;
#12009=PLANE('',#13732) ;
#12010=PLANE('',#13733) ;
#12011=PLANE('',#13741) ;
#12012=PLANE('',#13745) ;
#12013=PLANE('',#13748) ;
#12014=PLANE('',#13751) ;
#12015=PLANE('',#13752) ;
#12347=ADVANCED_FACE('',(#2952),#11995,.F.) ;
#12348=ADVANCED_FACE('',(#2953),#2673,.F.) ;
#12349=ADVANCED_FACE('',(#2954,#686),#2674,.F.) ;
#12350=ADVANCED_FACE('',(#2955),#2675,.F.) ;
#12351=ADVANCED_FACE('',(#2956),#11996,.F.) ;
#12352=ADVANCED_FACE('',(#2957,#687),#11997,.F.) ;
#12353=ADVANCED_FACE('',(#2958),#2676,.F.) ;
#12354=ADVANCED_FACE('',(#2959),#2677,.F.) ;
#12355=ADVANCED_FACE('',(#2960),#2678,.F.) ;
#12356=ADVANCED_FACE('',(#2961),#2679,.F.) ;
#12357=ADVANCED_FACE('',(#2962),#2680,.F.) ;
#12358=ADVANCED_FACE('',(#2963),#2681,.F.) ;
#12359=ADVANCED_FACE('',(#2964),#11998,.F.) ;
#12360=ADVANCED_FACE('',(#2965),#11999,.F.) ;
#12361=ADVANCED_FACE('',(#2966),#12000,.F.) ;
#12362=ADVANCED_FACE('',(#2967),#12001,.T.) ;
#12363=ADVANCED_FACE('',(#2968,#688,#689),#12002,.F.) ;
#12364=ADVANCED_FACE('',(#2969),#12003,.F.) ;
#12365=ADVANCED_FACE('',(#2970),#12004,.F.) ;
#12366=ADVANCED_FACE('',(#2971,#690),#2682,.T.) ;
#12367=ADVANCED_FACE('',(#2972),#2683,.F.) ;
#12368=ADVANCED_FACE('',(#2973),#2684,.T.) ;
#12369=ADVANCED_FACE('',(#2974),#2685,.T.) ;
#12370=ADVANCED_FACE('',(#2975,#691),#12005,.T.) ;
#12371=ADVANCED_FACE('',(#2976),#12006,.T.) ;
#12372=ADVANCED_FACE('',(#2977),#12007,.F.) ;
#12373=ADVANCED_FACE('',(#2978),#2686,.F.) ;
#12374=ADVANCED_FACE('',(#2979),#12008,.T.) ;
#12375=ADVANCED_FACE('',(#2980),#2687,.T.) ;
#12376=ADVANCED_FACE('',(#2981,#692),#12009,.T.) ;
#12377=ADVANCED_FACE('',(#2982,#693,#694,#695,#696,#697,#698,#699),#12010,
 .T.) ;
#12378=ADVANCED_FACE('',(#2983),#2688,.F.) ;
#12379=ADVANCED_FACE('',(#2984),#2689,.F.) ;
#12380=ADVANCED_FACE('',(#2985,#700),#12011,.F.) ;
#12381=ADVANCED_FACE('',(#2986),#2690,.F.) ;
#12382=ADVANCED_FACE('',(#2987,#701),#12012,.F.) ;
#12383=ADVANCED_FACE('',(#2988),#2691,.T.) ;
#12384=ADVANCED_FACE('',(#2989,#702),#12013,.T.) ;
#12385=ADVANCED_FACE('',(#2990),#2692,.T.) ;
#12386=ADVANCED_FACE('',(#2991,#703),#12014,.T.) ;
#12387=ADVANCED_FACE('',(#2992,#704,#705,#706,#707,#708,#709,#710),#12015,
 .T.) ;
#13114=CLOSED_SHELL('',(#12347,#12348,#12349,#12350,#12351,#12352,#12353,
#12354,#12355,#12356,#12357,#12358,#12359,#12360,#12361,#12362,#12363,#12364,
#12365,#12366,#12367,#12368,#12369,#12370,#12371,#12372,#12373,#12374,#12375,
#12376,#12377,#12378,#12379,#12380,#12381,#12382,#12383,#12384,#12385,#12386,
#12387)) ;
#13654=AXIS2_PLACEMENT_3D('',#19704,#15394,#15395) ;
#13655=AXIS2_PLACEMENT_3D('',#19705,#15396,#15397) ;
#13656=AXIS2_PLACEMENT_3D('',#19708,#15398,#15399) ;
#13657=AXIS2_PLACEMENT_3D('',#19710,#15400,#15401) ;
#13658=AXIS2_PLACEMENT_3D('',#19711,#15402,#15403) ;
#13659=AXIS2_PLACEMENT_3D('',#19712,#15404,#15405) ;
#13660=AXIS2_PLACEMENT_3D('',#19714,#15406,#15407) ;
#13661=AXIS2_PLACEMENT_3D('',#19719,#15410,#15411) ;
#13662=AXIS2_PLACEMENT_3D('',#19721,#15413,#15414) ;
#13663=AXIS2_PLACEMENT_3D('',#19723,#15415,#15416) ;
#13664=AXIS2_PLACEMENT_3D('',#19727,#15418,#15419) ;
#13665=AXIS2_PLACEMENT_3D('',#19731,#15421,#15422) ;
#13666=AXIS2_PLACEMENT_3D('',#19734,#15424,#15425) ;
#13667=AXIS2_PLACEMENT_3D('',#19736,#15426,#15427) ;
#13668=AXIS2_PLACEMENT_3D('',#19740,#15429,#15430) ;
#13669=AXIS2_PLACEMENT_3D('',#19743,#15432,#15433) ;
#13670=AXIS2_PLACEMENT_3D('',#19806,#15436,#15437) ;
#13671=AXIS2_PLACEMENT_3D('',#19808,#15438,#15439) ;
#13672=AXIS2_PLACEMENT_3D('',#19811,#15441,#15442) ;
#13673=AXIS2_PLACEMENT_3D('',#19812,#15443,#15444) ;
#13674=AXIS2_PLACEMENT_3D('',#19813,#15445,#15446) ;
#13675=AXIS2_PLACEMENT_3D('',#19814,#15447,#15448) ;
#13676=AXIS2_PLACEMENT_3D('',#19815,#15449,#15450) ;
#13677=AXIS2_PLACEMENT_3D('',#19817,#15451,#15452) ;
#13678=AXIS2_PLACEMENT_3D('',#19818,#15453,#15454) ;
#13679=AXIS2_PLACEMENT_3D('',#19820,#15455,#15456) ;
#13680=AXIS2_PLACEMENT_3D('',#19821,#15457,#15458) ;
#13681=AXIS2_PLACEMENT_3D('',#19823,#15459,#15460) ;
#13682=AXIS2_PLACEMENT_3D('',#19826,#15462,#15463) ;
#13683=AXIS2_PLACEMENT_3D('',#19827,#15464,#15465) ;
#13684=AXIS2_PLACEMENT_3D('',#19829,#15466,#15467) ;
#13685=AXIS2_PLACEMENT_3D('',#19832,#15469,#15470) ;
#13686=AXIS2_PLACEMENT_3D('',#19833,#15471,#15472) ;
#13687=AXIS2_PLACEMENT_3D('',#19835,#15473,#15474) ;
#13688=AXIS2_PLACEMENT_3D('',#19838,#15476,#15477) ;
#13689=AXIS2_PLACEMENT_3D('',#19839,#15478,#15479) ;
#13690=AXIS2_PLACEMENT_3D('',#19841,#15480,#15481) ;
#13691=AXIS2_PLACEMENT_3D('',#19844,#15483,#15484) ;
#13692=AXIS2_PLACEMENT_3D('',#19845,#15485,#15486) ;
#13693=AXIS2_PLACEMENT_3D('',#19847,#15487,#15488) ;
#13694=AXIS2_PLACEMENT_3D('',#19850,#15490,#15491) ;
#13695=AXIS2_PLACEMENT_3D('',#19851,#15492,#15493) ;
#13696=AXIS2_PLACEMENT_3D('',#19853,#15494,#15495) ;
#13697=AXIS2_PLACEMENT_3D('',#19856,#15497,#15498) ;
#13698=AXIS2_PLACEMENT_3D('',#19857,#15499,#15500) ;
#13699=AXIS2_PLACEMENT_3D('',#19870,#15507,#15508) ;
#13700=AXIS2_PLACEMENT_3D('',#19876,#15512,#15513) ;
#13701=AXIS2_PLACEMENT_3D('',#19878,#15514,#15515) ;
#13702=AXIS2_PLACEMENT_3D('',#19880,#15517,#15518) ;
#13703=AXIS2_PLACEMENT_3D('',#19886,#15522,#15523) ;
#13704=AXIS2_PLACEMENT_3D('',#19888,#15525,#15526) ;
#13705=AXIS2_PLACEMENT_3D('',#19890,#15527,#15528) ;
#13706=AXIS2_PLACEMENT_3D('',#19892,#15530,#15531) ;
#13707=AXIS2_PLACEMENT_3D('',#19896,#15534,#15535) ;
#13708=AXIS2_PLACEMENT_3D('',#19898,#15536,#15537) ;
#13709=AXIS2_PLACEMENT_3D('',#19901,#15539,#15540) ;
#13710=AXIS2_PLACEMENT_3D('',#19903,#15541,#15542) ;
#13711=AXIS2_PLACEMENT_3D('',#19907,#15544,#15545) ;
#13712=AXIS2_PLACEMENT_3D('',#19910,#15547,#15548) ;
#13713=AXIS2_PLACEMENT_3D('',#19965,#15549,#15550) ;
#13714=AXIS2_PLACEMENT_3D('',#19967,#15551,#15552) ;
#13715=AXIS2_PLACEMENT_3D('',#19969,#15554,#15555) ;
#13716=AXIS2_PLACEMENT_3D('',#19970,#15556,#15557) ;
#13717=AXIS2_PLACEMENT_3D('',#19973,#15559,#15560) ;
#13718=AXIS2_PLACEMENT_3D('',#19974,#15561,#15562) ;
#13719=AXIS2_PLACEMENT_3D('',#19975,#15563,#15564) ;
#13720=AXIS2_PLACEMENT_3D('',#19976,#15565,#15566) ;
#13721=AXIS2_PLACEMENT_3D('',#19977,#15567,#15568) ;
#13722=AXIS2_PLACEMENT_3D('',#19978,#15569,#15570) ;
#13723=AXIS2_PLACEMENT_3D('',#19979,#15571,#15572) ;
#13724=AXIS2_PLACEMENT_3D('',#19980,#15573,#15574) ;
#13725=AXIS2_PLACEMENT_3D('',#19982,#15575,#15576) ;
#13726=AXIS2_PLACEMENT_3D('',#19984,#15578,#15579) ;
#13727=AXIS2_PLACEMENT_3D('',#19985,#15580,#15581) ;
#13728=AXIS2_PLACEMENT_3D('',#19986,#15582,#15583) ;
#13729=AXIS2_PLACEMENT_3D('',#19988,#15584,#15585) ;
#13730=AXIS2_PLACEMENT_3D('',#19991,#15587,#15588) ;
#13731=AXIS2_PLACEMENT_3D('',#19992,#15589,#15590) ;
#13732=AXIS2_PLACEMENT_3D('',#19993,#15591,#15592) ;
#13733=AXIS2_PLACEMENT_3D('',#19994,#15593,#15594) ;
#13734=AXIS2_PLACEMENT_3D('',#19996,#15595,#15596) ;
#13735=AXIS2_PLACEMENT_3D('',#19997,#15597,#15598) ;
#13736=AXIS2_PLACEMENT_3D('',#19999,#15599,#15600) ;
#13737=AXIS2_PLACEMENT_3D('',#20002,#15602,#15603) ;
#13738=AXIS2_PLACEMENT_3D('',#20003,#15604,#15605) ;
#13739=AXIS2_PLACEMENT_3D('',#20005,#15606,#15607) ;
#13740=AXIS2_PLACEMENT_3D('',#20008,#15609,#15610) ;
#13741=AXIS2_PLACEMENT_3D('',#20009,#15611,#15612) ;
#13742=AXIS2_PLACEMENT_3D('',#20010,#15613,#15614) ;
#13743=AXIS2_PLACEMENT_3D('',#20012,#15615,#15616) ;
#13744=AXIS2_PLACEMENT_3D('',#20015,#15618,#15619) ;
#13745=AXIS2_PLACEMENT_3D('',#20016,#15620,#15621) ;
#13746=AXIS2_PLACEMENT_3D('',#20017,#15622,#15623) ;
#13747=AXIS2_PLACEMENT_3D('',#20019,#15624,#15625) ;
#13748=AXIS2_PLACEMENT_3D('',#20021,#15627,#15628) ;
#13749=AXIS2_PLACEMENT_3D('',#20022,#15629,#15630) ;
#13750=AXIS2_PLACEMENT_3D('',#20025,#15632,#15633) ;
#13751=AXIS2_PLACEMENT_3D('',#20026,#15634,#15635) ;
#13752=AXIS2_PLACEMENT_3D('',#20027,#15636,#15637) ;
#15394=DIRECTION('axis',(0.,0.,1.)) ;
#15395=DIRECTION('refdir',(1.,0.,0.)) ;
#15396=DIRECTION('center_axis',(0.,1.,0.)) ;
#15397=DIRECTION('ref_axis',(1.,0.,0.)) ;
#15398=DIRECTION('center_axis',(0.,-1.,0.)) ;
#15399=DIRECTION('ref_axis',(1.,0.,0.)) ;
#15400=DIRECTION('center_axis',(0.,1.,0.)) ;
#15401=DIRECTION('ref_axis',(1.,0.,0.)) ;
#15402=DIRECTION('center_axis',(0.,1.,0.)) ;
#15403=DIRECTION('ref_axis',(1.,0.,0.)) ;
#15404=DIRECTION('center_axis',(0.,1.,0.)) ;
#15405=DIRECTION('ref_axis',(1.,0.,0.)) ;
#15406=DIRECTION('center_axis',(0.,1.,0.)) ;
#15407=DIRECTION('ref_axis',(1.,0.,0.)) ;
#15408=DIRECTION('',(0.,1.,0.)) ;
#15409=DIRECTION('',(0.,1.,0.)) ;
#15410=DIRECTION('center_axis',(0.,-1.,0.)) ;
#15411=DIRECTION('ref_axis',(1.,0.,0.)) ;
#15412=DIRECTION('',(0.,-1.,0.)) ;
#15413=DIRECTION('center_axis',(0.,1.,0.)) ;
#15414=DIRECTION('ref_axis',(1.,0.,0.)) ;
#15415=DIRECTION('center_axis',(0.,-1.,0.)) ;
#15416=DIRECTION('ref_axis',(1.,0.,0.)) ;
#15417=DIRECTION('',(0.,1.,0.)) ;
#15418=DIRECTION('center_axis',(0.,-1.,0.)) ;
#15419=DIRECTION('ref_axis',(1.,0.,0.)) ;
#15420=DIRECTION('',(0.,-1.,0.)) ;
#15421=DIRECTION('center_axis',(0.,-1.,0.)) ;
#15422=DIRECTION('ref_axis',(1.,0.,0.)) ;
#15423=DIRECTION('',(0.,1.,0.)) ;
#15424=DIRECTION('center_axis',(0.,-1.,0.)) ;
#15425=DIRECTION('ref_axis',(1.,0.,0.)) ;
#15426=DIRECTION('center_axis',(0.,-1.,0.)) ;
#15427=DIRECTION('ref_axis',(1.,0.,0.)) ;
#15428=DIRECTION('',(0.,1.,0.)) ;
#15429=DIRECTION('center_axis',(0.,-1.,0.)) ;
#15430=DIRECTION('ref_axis',(1.,0.,0.)) ;
#15431=DIRECTION('',(0.,-1.,0.)) ;
#15432=DIRECTION('center_axis',(0.,-1.,0.)) ;
#15433=DIRECTION('ref_axis',(1.,0.,0.)) ;
#15434=DIRECTION('',(0.,1.,0.)) ;
#15435=DIRECTION('',(0.,1.,0.)) ;
#15436=DIRECTION('center_axis',(0.,1.,0.)) ;
#15437=DIRECTION('ref_axis',(1.,0.,0.)) ;
#15438=DIRECTION('center_axis',(0.,1.,0.)) ;
#15439=DIRECTION('ref_axis',(1.,0.,0.)) ;
#15440=DIRECTION('',(0.,1.,0.)) ;
#15441=DIRECTION('center_axis',(0.,1.,0.)) ;
#15442=DIRECTION('ref_axis',(1.,0.,0.)) ;
#15443=DIRECTION('center_axis',(0.,-1.,0.)) ;
#15444=DIRECTION('ref_axis',(1.,0.,0.)) ;
#15445=DIRECTION('center_axis',(0.,1.,0.)) ;
#15446=DIRECTION('ref_axis',(1.,0.,0.)) ;
#15447=DIRECTION('center_axis',(0.,1.,0.)) ;
#15448=DIRECTION('ref_axis',(1.,0.,0.)) ;
#15449=DIRECTION('center_axis',(0.,-1.,0.)) ;
#15450=DIRECTION('ref_axis',(-1.,0.,0.)) ;
#15451=DIRECTION('center_axis',(0.,-1.,0.)) ;
#15452=DIRECTION('ref_axis',(1.,0.,0.)) ;
#15453=DIRECTION('center_axis',(0.,-1.,0.)) ;
#15454=DIRECTION('ref_axis',(1.,0.,0.)) ;
#15455=DIRECTION('center_axis',(0.,-1.,0.)) ;
#15456=DIRECTION('ref_axis',(1.,0.,0.)) ;
#15457=DIRECTION('center_axis',(0.,1.,0.)) ;
#15458=DIRECTION('ref_axis',(1.,0.,0.)) ;
#15459=DIRECTION('center_axis',(0.,1.,0.)) ;
#15460=DIRECTION('ref_axis',(1.,0.,0.)) ;
#15461=DIRECTION('',(0.,1.,0.)) ;
#15462=DIRECTION('center_axis',(0.,-1.,0.)) ;
#15463=DIRECTION('ref_axis',(1.,0.,0.)) ;
#15464=DIRECTION('center_axis',(0.,1.,0.)) ;
#15465=DIRECTION('ref_axis',(1.,0.,0.)) ;
#15466=DIRECTION('center_axis',(0.,1.,0.)) ;
#15467=DIRECTION('ref_axis',(1.,0.,0.)) ;
#15468=DIRECTION('',(0.,1.,0.)) ;
#15469=DIRECTION('center_axis',(0.,-1.,0.)) ;
#15470=DIRECTION('ref_axis',(1.,0.,0.)) ;
#15471=DIRECTION('center_axis',(0.,1.,0.)) ;
#15472=DIRECTION('ref_axis',(1.,0.,0.)) ;
#15473=DIRECTION('center_axis',(0.,1.,0.)) ;
#15474=DIRECTION('ref_axis',(1.,0.,0.)) ;
#15475=DIRECTION('',(0.,1.,0.)) ;
#15476=DIRECTION('center_axis',(0.,-1.,0.)) ;
#15477=DIRECTION('ref_axis',(1.,0.,0.)) ;
#15478=DIRECTION('center_axis',(0.,1.,0.)) ;
#15479=DIRECTION('ref_axis',(1.,0.,0.)) ;
#15480=DIRECTION('center_axis',(0.,1.,0.)) ;
#15481=DIRECTION('ref_axis',(1.,0.,0.)) ;
#15482=DIRECTION('',(0.,1.,0.)) ;
#15483=DIRECTION('center_axis',(0.,-1.,0.)) ;
#15484=DIRECTION('ref_axis',(1.,0.,0.)) ;
#15485=DIRECTION('center_axis',(0.,1.,0.)) ;
#15486=DIRECTION('ref_axis',(1.,0.,0.)) ;
#15487=DIRECTION('center_axis',(0.,1.,0.)) ;
#15488=DIRECTION('ref_axis',(1.,0.,0.)) ;
#15489=DIRECTION('',(0.,1.,0.)) ;
#15490=DIRECTION('center_axis',(0.,-1.,0.)) ;
#15491=DIRECTION('ref_axis',(1.,0.,0.)) ;
#15492=DIRECTION('center_axis',(0.,1.,0.)) ;
#15493=DIRECTION('ref_axis',(1.,0.,0.)) ;
#15494=DIRECTION('center_axis',(0.,1.,0.)) ;
#15495=DIRECTION('ref_axis',(1.,0.,0.)) ;
#15496=DIRECTION('',(0.,1.,0.)) ;
#15497=DIRECTION('center_axis',(0.,-1.,0.)) ;
#15498=DIRECTION('ref_axis',(1.,0.,0.)) ;
#15499=DIRECTION('center_axis',(1.,0.,0.)) ;
#15500=DIRECTION('ref_axis',(0.,0.,-1.)) ;
#15501=DIRECTION('',(0.,1.,0.)) ;
#15502=DIRECTION('',(0.,0.,1.)) ;
#15503=DIRECTION('',(0.,1.,0.)) ;
#15504=DIRECTION('',(0.,0.,-1.)) ;
#15505=DIRECTION('',(0.,-1.,0.)) ;
#15506=DIRECTION('',(0.,0.,-1.)) ;
#15507=DIRECTION('center_axis',(0.,0.,1.)) ;
#15508=DIRECTION('ref_axis',(1.,0.,0.)) ;
#15509=DIRECTION('',(-1.,0.,0.)) ;
#15510=DIRECTION('',(0.,-1.,0.)) ;
#15511=DIRECTION('',(-1.,0.,0.)) ;
#15512=DIRECTION('center_axis',(0.,-1.,0.)) ;
#15513=DIRECTION('ref_axis',(0.,0.,-1.)) ;
#15514=DIRECTION('center_axis',(0.,1.,0.)) ;
#15515=DIRECTION('ref_axis',(1.,0.,0.)) ;
#15516=DIRECTION('',(-1.,0.,0.)) ;
#15517=DIRECTION('center_axis',(0.,0.,1.)) ;
#15518=DIRECTION('ref_axis',(1.,0.,0.)) ;
#15519=DIRECTION('',(0.,1.,0.)) ;
#15520=DIRECTION('',(-1.,0.,0.)) ;
#15521=DIRECTION('',(1.,0.,0.)) ;
#15522=DIRECTION('center_axis',(0.,1.,0.)) ;
#15523=DIRECTION('ref_axis',(0.,0.,1.)) ;
#15524=DIRECTION('',(0.,0.,-1.)) ;
#15525=DIRECTION('center_axis',(0.,-1.,0.)) ;
#15526=DIRECTION('ref_axis',(0.,0.,-1.)) ;
#15527=DIRECTION('center_axis',(0.,1.,0.)) ;
#15528=DIRECTION('ref_axis',(1.,0.,0.)) ;
#15529=DIRECTION('',(0.,0.,-1.)) ;
#15530=DIRECTION('center_axis',(-1.,0.,0.)) ;
#15531=DIRECTION('ref_axis',(0.,0.,1.)) ;
#15532=DIRECTION('',(0.,-1.,0.)) ;
#15533=DIRECTION('',(0.,0.,-1.)) ;
#15534=DIRECTION('center_axis',(0.,1.,0.)) ;
#15535=DIRECTION('ref_axis',(1.,0.,0.)) ;
#15536=DIRECTION('center_axis',(0.,1.,0.)) ;
#15537=DIRECTION('ref_axis',(1.,0.,0.)) ;
#15538=DIRECTION('',(0.,-1.,0.)) ;
#15539=DIRECTION('center_axis',(0.,-1.,0.)) ;
#15540=DIRECTION('ref_axis',(1.,0.,0.)) ;
#15541=DIRECTION('center_axis',(0.,-1.,0.)) ;
#15542=DIRECTION('ref_axis',(1.,0.,0.)) ;
#15543=DIRECTION('',(0.,1.,0.)) ;
#15544=DIRECTION('center_axis',(0.,1.,0.)) ;
#15545=DIRECTION('ref_axis',(1.,0.,0.)) ;
#15546=DIRECTION('',(0.,-1.,0.)) ;
#15547=DIRECTION('center_axis',(0.,-1.,0.)) ;
#15548=DIRECTION('ref_axis',(1.,0.,0.)) ;
#15549=DIRECTION('center_axis',(0.,0.,1.)) ;
#15550=DIRECTION('ref_axis',(1.,0.,0.)) ;
#15551=DIRECTION('center_axis',(0.,0.,1.)) ;
#15552=DIRECTION('ref_axis',(1.,0.,0.)) ;
#15553=DIRECTION('',(0.,0.,1.)) ;
#15554=DIRECTION('center_axis',(0.,0.,-1.)) ;
#15555=DIRECTION('ref_axis',(1.,0.,0.)) ;
#15556=DIRECTION('center_axis',(0.,0.,1.)) ;
#15557=DIRECTION('ref_axis',(1.,0.,0.)) ;
#15558=DIRECTION('',(0.,0.,-1.)) ;
#15559=DIRECTION('center_axis',(0.,0.,-1.)) ;
#15560=DIRECTION('ref_axis',(1.,0.,0.)) ;
#15561=DIRECTION('center_axis',(0.,0.,1.)) ;
#15562=DIRECTION('ref_axis',(1.,0.,0.)) ;
#15563=DIRECTION('center_axis',(0.,0.,1.)) ;
#15564=DIRECTION('ref_axis',(1.,0.,0.)) ;
#15565=DIRECTION('center_axis',(0.,0.,-1.)) ;
#15566=DIRECTION('ref_axis',(-1.,0.,0.)) ;
#15567=DIRECTION('center_axis',(0.,0.,1.)) ;
#15568=DIRECTION('ref_axis',(1.,0.,0.)) ;
#15569=DIRECTION('center_axis',(0.,1.,0.)) ;
#15570=DIRECTION('ref_axis',(1.,0.,0.)) ;
#15571=DIRECTION('center_axis',(0.,1.,0.)) ;
#15572=DIRECTION('ref_axis',(1.,0.,0.)) ;
#15573=DIRECTION('center_axis',(0.,1.,0.)) ;
#15574=DIRECTION('ref_axis',(1.,0.,0.)) ;
#15575=DIRECTION('center_axis',(0.,1.,0.)) ;
#15576=DIRECTION('ref_axis',(1.,0.,0.)) ;
#15577=DIRECTION('',(0.,1.,0.)) ;
#15578=DIRECTION('center_axis',(0.,1.,0.)) ;
#15579=DIRECTION('ref_axis',(1.,0.,0.)) ;
#15580=DIRECTION('center_axis',(0.,1.,0.)) ;
#15581=DIRECTION('ref_axis',(1.,0.,0.)) ;
#15582=DIRECTION('center_axis',(0.,1.,0.)) ;
#15583=DIRECTION('ref_axis',(1.,0.,0.)) ;
#15584=DIRECTION('center_axis',(0.,1.,0.)) ;
#15585=DIRECTION('ref_axis',(1.,0.,0.)) ;
#15586=DIRECTION('',(0.,-1.,0.)) ;
#15587=DIRECTION('center_axis',(0.,-1.,0.)) ;
#15588=DIRECTION('ref_axis',(1.,0.,0.)) ;
#15589=DIRECTION('center_axis',(0.,1.,0.)) ;
#15590=DIRECTION('ref_axis',(1.,0.,0.)) ;
#15591=DIRECTION('center_axis',(0.,-1.,0.)) ;
#15592=DIRECTION('ref_axis',(-1.,0.,0.)) ;
#15593=DIRECTION('center_axis',(0.,-1.,0.)) ;
#15594=DIRECTION('ref_axis',(-1.,0.,0.)) ;
#15595=DIRECTION('center_axis',(0.,1.,0.)) ;
#15596=DIRECTION('ref_axis',(1.,0.,0.)) ;
#15597=DIRECTION('center_axis',(0.,1.,0.)) ;
#15598=DIRECTION('ref_axis',(1.,0.,0.)) ;
#15599=DIRECTION('center_axis',(0.,1.,0.)) ;
#15600=DIRECTION('ref_axis',(1.,0.,0.)) ;
#15601=DIRECTION('',(0.,1.,0.)) ;
#15602=DIRECTION('center_axis',(0.,-1.,0.)) ;
#15603=DIRECTION('ref_axis',(1.,0.,0.)) ;
#15604=DIRECTION('center_axis',(0.,1.,0.)) ;
#15605=DIRECTION('ref_axis',(1.,0.,0.)) ;
#15606=DIRECTION('center_axis',(0.,-1.,0.)) ;
#15607=DIRECTION('ref_axis',(1.,0.,0.)) ;
#15608=DIRECTION('',(0.,1.,0.)) ;
#15609=DIRECTION('center_axis',(0.,-1.,0.)) ;
#15610=DIRECTION('ref_axis',(1.,0.,0.)) ;
#15611=DIRECTION('center_axis',(0.,-1.,0.)) ;
#15612=DIRECTION('ref_axis',(-1.,0.,0.)) ;
#15613=DIRECTION('center_axis',(0.,1.,0.)) ;
#15614=DIRECTION('ref_axis',(1.,0.,0.)) ;
#15615=DIRECTION('center_axis',(0.,1.,0.)) ;
#15616=DIRECTION('ref_axis',(1.,0.,0.)) ;
#15617=DIRECTION('',(0.,1.,0.)) ;
#15618=DIRECTION('center_axis',(0.,1.,0.)) ;
#15619=DIRECTION('ref_axis',(1.,0.,0.)) ;
#15620=DIRECTION('center_axis',(0.,1.,0.)) ;
#15621=DIRECTION('ref_axis',(1.,0.,0.)) ;
#15622=DIRECTION('center_axis',(0.,1.,0.)) ;
#15623=DIRECTION('ref_axis',(1.,0.,0.)) ;
#15624=DIRECTION('center_axis',(0.,1.,0.)) ;
#15625=DIRECTION('ref_axis',(1.,0.,0.)) ;
#15626=DIRECTION('',(0.,-1.,0.)) ;
#15627=DIRECTION('center_axis',(0.,1.,0.)) ;
#15628=DIRECTION('ref_axis',(1.,0.,0.)) ;
#15629=DIRECTION('center_axis',(0.,1.,0.)) ;
#15630=DIRECTION('ref_axis',(1.,0.,0.)) ;
#15631=DIRECTION('',(0.,-1.,0.)) ;
#15632=DIRECTION('center_axis',(0.,-1.,0.)) ;
#15633=DIRECTION('ref_axis',(1.,0.,0.)) ;
#15634=DIRECTION('center_axis',(0.,-1.,0.)) ;
#15635=DIRECTION('ref_axis',(-1.,0.,0.)) ;
#15636=DIRECTION('center_axis',(0.,1.,0.)) ;
#15637=DIRECTION('ref_axis',(1.,0.,0.)) ;
#19704=CARTESIAN_POINT('',(0.,0.,0.)) ;
#19705=CARTESIAN_POINT('Origin',(2.5,-3.5,11.5)) ;
#19706=CARTESIAN_POINT('',(2.59406867944788,-3.5,11.1009372435983)) ;
#19707=CARTESIAN_POINT('',(2.24874539997451,-3.5,11.1760075217447)) ;
#19708=CARTESIAN_POINT('Origin',(0.,-3.5,0.)) ;
#19709=CARTESIAN_POINT('',(2.09,-3.5,11.5)) ;
#19710=CARTESIAN_POINT('Origin',(2.5,-3.5,11.5)) ;
#19711=CARTESIAN_POINT('Origin',(2.5,-3.5,11.5)) ;
#19712=CARTESIAN_POINT('Origin',(2.5,-4.1,11.5)) ;
#19713=CARTESIAN_POINT('',(2.09,-4.6,11.5)) ;
#19714=CARTESIAN_POINT('Origin',(2.5,-4.6,11.5)) ;
#19715=CARTESIAN_POINT('',(2.09,-4.1,11.5)) ;
#19716=CARTESIAN_POINT('',(2.59406867944801,-3.6,11.1009372435983)) ;
#19717=CARTESIAN_POINT('',(2.59406867944788,-4.1,11.1009372435983)) ;
#19718=CARTESIAN_POINT('',(2.24874539997437,-3.6,11.1760075217447)) ;
#19719=CARTESIAN_POINT('Origin',(2.5,-3.6,11.5)) ;
#19720=CARTESIAN_POINT('',(2.24874539997451,-4.1,11.1760075217447)) ;
#19721=CARTESIAN_POINT('Origin',(0.,-1.8,0.)) ;
#19722=CARTESIAN_POINT('',(-2.24874539997437,-3.6,11.1760075217447)) ;
#19723=CARTESIAN_POINT('Origin',(0.,-3.6,0.)) ;
#19724=CARTESIAN_POINT('',(-2.24874539997451,-3.5,11.1760075217447)) ;
#19725=CARTESIAN_POINT('',(-2.24874539997451,-4.1,11.1760075217447)) ;
#19726=CARTESIAN_POINT('',(-2.59406867944788,-3.5,11.1009372435983)) ;
#19727=CARTESIAN_POINT('Origin',(0.,-3.5,0.)) ;
#19728=CARTESIAN_POINT('',(-2.59406867944801,-3.6,11.1009372435983)) ;
#19729=CARTESIAN_POINT('',(-2.59406867944788,-4.1,11.1009372435983)) ;
#19730=CARTESIAN_POINT('',(-11.4,-3.6,1.39609735102798E-15)) ;
#19731=CARTESIAN_POINT('Origin',(0.,-3.6,0.)) ;
#19732=CARTESIAN_POINT('',(-11.4,-0.0999999999999999,-1.39609735102798E-15)) ;
#19733=CARTESIAN_POINT('',(-11.4,-1.8,1.39609735102798E-15)) ;
#19734=CARTESIAN_POINT('Origin',(0.,-0.0999999999999999,0.)) ;
#19735=CARTESIAN_POINT('',(7.40055690846941,-3.6,-8.67131809153059)) ;
#19736=CARTESIAN_POINT('Origin',(0.,-3.6,0.)) ;
#19737=CARTESIAN_POINT('',(7.40055690846942,-3.,-8.67131809153058)) ;
#19738=CARTESIAN_POINT('',(7.40055690846942,-4.65,-8.67131809153058)) ;
#19739=CARTESIAN_POINT('',(8.67131809153058,-3.,-7.40055690846942)) ;
#19740=CARTESIAN_POINT('Origin',(0.,-3.,0.)) ;
#19741=CARTESIAN_POINT('',(8.67131809153059,-3.6,-7.40055690846941)) ;
#19742=CARTESIAN_POINT('',(8.67131809153058,-4.65,-7.40055690846942)) ;
#19743=CARTESIAN_POINT('Origin',(0.,-3.6,0.)) ;
#19744=CARTESIAN_POINT('',(-2.12602916254692,-2.46796330384352,-11.2)) ;
#19745=CARTESIAN_POINT('',(-4.1,-1.8,-10.6371988794043)) ;
#19746=CARTESIAN_POINT('Ctrl Pts',(-2.12602916254691,-2.46796330384352,
-11.2)) ;
#19747=CARTESIAN_POINT('Ctrl Pts',(-2.15513164480001,-2.50604132495688,
-11.1944756494667)) ;
#19748=CARTESIAN_POINT('Ctrl Pts',(-2.18630985484209,-2.54164208401901,
-11.1884379436503)) ;
#19749=CARTESIAN_POINT('Ctrl Pts',(-2.31779618826562,-2.67429360771505,
-11.1623481119451)) ;
#19750=CARTESIAN_POINT('Ctrl Pts',(-2.44303520251314,-2.75997478721919,
-11.1360298274263)) ;
#19751=CARTESIAN_POINT('Ctrl Pts',(-2.71564409591941,-2.87280151063408,
-11.0727078200836)) ;
#19752=CARTESIAN_POINT('Ctrl Pts',(-2.86295917531106,-2.9,-11.0355626174438)) ;
#19753=CARTESIAN_POINT('Ctrl Pts',(-3.13999995839577,-2.9,-10.9599935484512)) ;
#19754=CARTESIAN_POINT('Ctrl Pts',(-3.28870394625325,-2.87173395468652,
-10.9162703933172)) ;
#19755=CARTESIAN_POINT('Ctrl Pts',(-3.5620474526488,-2.75711351549606,-10.8301593198666)) ;
#19756=CARTESIAN_POINT('Ctrl Pts',(-3.68673548477559,-2.67077361394648,
-10.787906168642)) ;
#19757=CARTESIAN_POINT('Ctrl Pts',(-3.87930809485592,-2.47439729417,-10.7201158159833)) ;
#19758=CARTESIAN_POINT('Ctrl Pts',(-3.96197425311411,-2.35282868058528,
-10.6895386999817)) ;
#19759=CARTESIAN_POINT('Ctrl Pts',(-4.07235177185144,-2.08473780880403,
-10.6479776813726)) ;
#19760=CARTESIAN_POINT('Ctrl Pts',(-4.1,-1.93815780811578,-10.6371988794043)) ;
#19761=CARTESIAN_POINT('Ctrl Pts',(-4.1,-1.8,-10.6371988794043)) ;
#19762=CARTESIAN_POINT('',(-2.12602916254692,-1.13203669615648,-11.2)) ;
#19763=CARTESIAN_POINT('Ctrl Pts',(-4.1,-1.8,-10.6371988794043)) ;
#19764=CARTESIAN_POINT('Ctrl Pts',(-4.1,-1.66184219188422,-10.6371988794043)) ;
#19765=CARTESIAN_POINT('Ctrl Pts',(-4.07235177185144,-1.51526219119597,
-10.6479776813726)) ;
#19766=CARTESIAN_POINT('Ctrl Pts',(-3.9619742531141,-1.24717131941471,-10.6895386999817)) ;
#19767=CARTESIAN_POINT('Ctrl Pts',(-3.87930809485592,-1.12560270583,-10.7201158159833)) ;
#19768=CARTESIAN_POINT('Ctrl Pts',(-3.68673548477559,-0.929226386053517,
-10.787906168642)) ;
#19769=CARTESIAN_POINT('Ctrl Pts',(-3.5620474526488,-0.842886484503946,
-10.8301593198666)) ;
#19770=CARTESIAN_POINT('Ctrl Pts',(-3.28870394625325,-0.728266045313485,
-10.9162703933172)) ;
#19771=CARTESIAN_POINT('Ctrl Pts',(-3.13999995839577,-0.7,-10.9599935484512)) ;
#19772=CARTESIAN_POINT('Ctrl Pts',(-2.86295917531106,-0.7,-11.0355626174438)) ;
#19773=CARTESIAN_POINT('Ctrl Pts',(-2.71564409591941,-0.727198489365921,
-11.0727078200836)) ;
#19774=CARTESIAN_POINT('Ctrl Pts',(-2.44303520251314,-0.840025212780807,
-11.1360298274263)) ;
#19775=CARTESIAN_POINT('Ctrl Pts',(-2.31779618826562,-0.925706392284951,
-11.1623481119451)) ;
#19776=CARTESIAN_POINT('Ctrl Pts',(-2.18630985484209,-1.05835791598098,
-11.1884379436503)) ;
#19777=CARTESIAN_POINT('Ctrl Pts',(-2.15513164480001,-1.09395867504312,
-11.1944756494667)) ;
#19778=CARTESIAN_POINT('Ctrl Pts',(-2.12602916254692,-1.13203669615648,
-11.2)) ;
#19779=CARTESIAN_POINT('',(-2.12602916254692,-0.580912236431864,-11.2)) ;
#19780=CARTESIAN_POINT('',(-2.12602916254692,-1.8,-11.2)) ;
#19781=CARTESIAN_POINT('',(-2.12602916254692,-3.01908776356814,-11.2)) ;
#19782=CARTESIAN_POINT('Ctrl Pts',(-2.12602916254692,-0.580912236431864,
-11.2)) ;
#19783=CARTESIAN_POINT('Ctrl Pts',(-2.05711563629085,-0.63031672891695,
-11.2130814434388)) ;
#19784=CARTESIAN_POINT('Ctrl Pts',(-1.99323281619767,-0.685058529370311,
-11.2245461145188)) ;
#19785=CARTESIAN_POINT('Ctrl Pts',(-1.86992093614613,-0.809229549581467,
-11.2457923763132)) ;
#19786=CARTESIAN_POINT('Ctrl Pts',(-1.80806979456003,-0.88406833950675,
-11.2558400434588)) ;
#19787=CARTESIAN_POINT('Ctrl Pts',(-1.69890438988511,-1.04715298044695,
-11.2728335098074)) ;
#19788=CARTESIAN_POINT('Ctrl Pts',(-1.6515851116445,-1.13539399284769,-11.2797935238811)) ;
#19789=CARTESIAN_POINT('Ctrl Pts',(-1.575538988389,-1.31954738708738,-11.2906665964395)) ;
#19790=CARTESIAN_POINT('Ctrl Pts',(-1.54675013780201,-1.41560915257294,
-11.2945972589809)) ;
#19791=CARTESIAN_POINT('Ctrl Pts',(-1.50897676604781,-1.6088424695419,-11.2997058524029)) ;
#19792=CARTESIAN_POINT('Ctrl Pts',(-1.5,-1.70601550683761,-11.3008849211024)) ;
#19793=CARTESIAN_POINT('Ctrl Pts',(-1.5,-1.8,-11.3008849211024)) ;
#19794=CARTESIAN_POINT('Ctrl Pts',(-1.5,-1.89398449316239,-11.3008849211024)) ;
#19795=CARTESIAN_POINT('Ctrl Pts',(-1.50897676604781,-1.9911575304581,-11.2997058524029)) ;
#19796=CARTESIAN_POINT('Ctrl Pts',(-1.54675013780201,-2.18439084742706,
-11.2945972589809)) ;
#19797=CARTESIAN_POINT('Ctrl Pts',(-1.575538988389,-2.28045261291263,-11.2906665964395)) ;
#19798=CARTESIAN_POINT('Ctrl Pts',(-1.6515851116445,-2.46460600715231,-11.2797935238811)) ;
#19799=CARTESIAN_POINT('Ctrl Pts',(-1.69890438988511,-2.55284701955305,
-11.2728335098074)) ;
#19800=CARTESIAN_POINT('Ctrl Pts',(-1.80806979456003,-2.71593166049325,
-11.2558400434588)) ;
#19801=CARTESIAN_POINT('Ctrl Pts',(-1.86992093614613,-2.79077045041853,
-11.2457923763132)) ;
#19802=CARTESIAN_POINT('Ctrl Pts',(-1.99323281619761,-2.91494147062963,
-11.2245461145188)) ;
#19803=CARTESIAN_POINT('Ctrl Pts',(-2.05711563629117,-2.96968327108328,
-11.2130814434387)) ;
#19804=CARTESIAN_POINT('Ctrl Pts',(-2.12602916254692,-3.01908776356814,
-11.2)) ;
#19805=CARTESIAN_POINT('',(-2.12602916254692,-1.8,-11.2)) ;
#19806=CARTESIAN_POINT('Origin',(-2.5,-4.1,11.5)) ;
#19807=CARTESIAN_POINT('',(-2.91,-4.6,11.5)) ;
#19808=CARTESIAN_POINT('Origin',(-2.5,-4.6,11.5)) ;
#19809=CARTESIAN_POINT('',(-2.91,-3.5,11.5)) ;
#19810=CARTESIAN_POINT('',(-2.91,-4.1,11.5)) ;
#19811=CARTESIAN_POINT('Origin',(-2.5,-3.5,11.5)) ;
#19812=CARTESIAN_POINT('Origin',(-2.5,-3.6,11.5)) ;
#19813=CARTESIAN_POINT('Origin',(-2.5,-3.5,11.5)) ;
#19814=CARTESIAN_POINT('Origin',(-2.5,-3.5,11.5)) ;
#19815=CARTESIAN_POINT('Origin',(0.,-3.6,0.)) ;
#19816=CARTESIAN_POINT('',(7.1,-3.6,-8.)) ;
#19817=CARTESIAN_POINT('Origin',(8.,-3.6,-8.)) ;
#19818=CARTESIAN_POINT('Origin',(8.,-3.6,-8.)) ;
#19819=CARTESIAN_POINT('',(-2.5,-3.6,3.06161699786838E-16)) ;
#19820=CARTESIAN_POINT('Origin',(0.,-3.6,0.)) ;
#19821=CARTESIAN_POINT('Origin',(5.975,-2.,-10.349003575224)) ;
#19822=CARTESIAN_POINT('',(5.65,-4.,-10.349003575224)) ;
#19823=CARTESIAN_POINT('Origin',(5.975,-4.,-10.349003575224)) ;
#19824=CARTESIAN_POINT('',(5.65,-0.0999999999999999,-10.349003575224)) ;
#19825=CARTESIAN_POINT('',(5.65,-2.,-10.349003575224)) ;
#19826=CARTESIAN_POINT('Origin',(5.975,-0.0999999999999999,-10.349003575224)) ;
#19827=CARTESIAN_POINT('Origin',(-5.975,-2.,-10.349003575224)) ;
#19828=CARTESIAN_POINT('',(-6.30000000000001,-4.,-10.349003575224)) ;
#19829=CARTESIAN_POINT('Origin',(-5.975,-4.,-10.349003575224)) ;
#19830=CARTESIAN_POINT('',(-6.30000000000001,-0.0999999999999999,-10.349003575224)) ;
#19831=CARTESIAN_POINT('',(-6.30000000000001,-2.,-10.349003575224)) ;
#19832=CARTESIAN_POINT('Origin',(-5.975,-0.0999999999999999,-10.349003575224)) ;
#19833=CARTESIAN_POINT('Origin',(-11.95,-2.,1.46345292498109E-15)) ;
#19834=CARTESIAN_POINT('',(-12.275,-4.,1.50325394595338E-15)) ;
#19835=CARTESIAN_POINT('Origin',(-11.95,-4.,1.46345292498109E-15)) ;
#19836=CARTESIAN_POINT('',(-12.275,-0.0999999999999999,1.4236519040088E-15)) ;
#19837=CARTESIAN_POINT('',(-12.275,-2.,1.50325394595338E-15)) ;
#19838=CARTESIAN_POINT('Origin',(-11.95,-0.0999999999999999,1.46345292498109E-15)) ;
#19839=CARTESIAN_POINT('Origin',(-5.975,-2.,10.349003575224)) ;
#19840=CARTESIAN_POINT('',(-6.3,-4.,10.349003575224)) ;
#19841=CARTESIAN_POINT('Origin',(-5.975,-4.,10.349003575224)) ;
#19842=CARTESIAN_POINT('',(-6.3,-0.0999999999999999,10.349003575224)) ;
#19843=CARTESIAN_POINT('',(-6.3,-2.,10.349003575224)) ;
#19844=CARTESIAN_POINT('Origin',(-5.975,-0.0999999999999999,10.349003575224)) ;
#19845=CARTESIAN_POINT('Origin',(5.975,-2.,10.349003575224)) ;
#19846=CARTESIAN_POINT('',(5.65,-4.,10.349003575224)) ;
#19847=CARTESIAN_POINT('Origin',(5.975,-4.,10.349003575224)) ;
#19848=CARTESIAN_POINT('',(5.65,-0.0999999999999999,10.349003575224)) ;
#19849=CARTESIAN_POINT('',(5.65,-2.,10.349003575224)) ;
#19850=CARTESIAN_POINT('Origin',(5.975,-0.0999999999999999,10.349003575224)) ;
#19851=CARTESIAN_POINT('Origin',(11.95,-2.,0.)) ;
#19852=CARTESIAN_POINT('',(11.625,-4.,3.9801020972289E-17)) ;
#19853=CARTESIAN_POINT('Origin',(11.95,-4.,0.)) ;
#19854=CARTESIAN_POINT('',(11.625,-0.0999999999999999,-3.9801020972289E-17)) ;
#19855=CARTESIAN_POINT('',(11.625,-2.,3.9801020972289E-17)) ;
#19856=CARTESIAN_POINT('Origin',(11.95,-0.0999999999999999,0.)) ;
#19857=CARTESIAN_POINT('Origin',(-4.,-4.1,11.25)) ;
#19858=CARTESIAN_POINT('',(-4.,-4.,11.842719282327)) ;
#19859=CARTESIAN_POINT('',(-4.,-3.6,11.842719282327)) ;
#19860=CARTESIAN_POINT('',(-4.,-2.05,11.842719282327)) ;
#19861=CARTESIAN_POINT('',(-4.,-4.,10.)) ;
#19862=CARTESIAN_POINT('',(-4.,-4.,5.625)) ;
#19863=CARTESIAN_POINT('',(-4.,-4.6,10.)) ;
#19864=CARTESIAN_POINT('',(-4.,-4.1,10.)) ;
#19865=CARTESIAN_POINT('',(-4.,-4.6,12.5)) ;
#19866=CARTESIAN_POINT('',(-4.,-4.6,11.25)) ;
#19867=CARTESIAN_POINT('',(-4.,-3.6,12.5)) ;
#19868=CARTESIAN_POINT('',(-4.,-4.1,12.5)) ;
#19869=CARTESIAN_POINT('',(-4.,-3.6,11.25)) ;
#19870=CARTESIAN_POINT('Origin',(0.,-4.1,10.)) ;
#19871=CARTESIAN_POINT('',(4.,-4.,10.)) ;
#19872=CARTESIAN_POINT('',(0.,-4.,10.)) ;
#19873=CARTESIAN_POINT('',(4.,-4.6,10.)) ;
#19874=CARTESIAN_POINT('',(4.,-4.1,10.)) ;
#19875=CARTESIAN_POINT('',(0.,-4.6,10.)) ;
#19876=CARTESIAN_POINT('Origin',(0.,-3.6,11.25)) ;
#19877=CARTESIAN_POINT('',(0.,-3.6,12.5)) ;
#19878=CARTESIAN_POINT('Origin',(0.,-3.6,0.)) ;
#19879=CARTESIAN_POINT('',(0.,-3.6,12.5)) ;
#19880=CARTESIAN_POINT('Origin',(0.,-4.1,12.5)) ;
#19881=CARTESIAN_POINT('',(4.,-4.6,12.5)) ;
#19882=CARTESIAN_POINT('',(4.,-3.6,12.5)) ;
#19883=CARTESIAN_POINT('',(4.,-4.1,12.5)) ;
#19884=CARTESIAN_POINT('',(0.,-3.6,12.5)) ;
#19885=CARTESIAN_POINT('',(0.,-4.6,12.5)) ;
#19886=CARTESIAN_POINT('Origin',(0.,-4.6,11.25)) ;
#19887=CARTESIAN_POINT('',(4.,-4.6,11.25)) ;
#19888=CARTESIAN_POINT('Origin',(0.,-3.6,11.25)) ;
#19889=CARTESIAN_POINT('',(4.,-3.6,11.842719282327)) ;
#19890=CARTESIAN_POINT('Origin',(0.,-3.6,0.)) ;
#19891=CARTESIAN_POINT('',(4.,-3.6,11.25)) ;
#19892=CARTESIAN_POINT('Origin',(4.,-4.1,11.25)) ;
#19893=CARTESIAN_POINT('',(4.,-4.,11.842719282327)) ;
#19894=CARTESIAN_POINT('',(4.,-2.05,11.842719282327)) ;
#19895=CARTESIAN_POINT('',(4.,-4.,5.625)) ;
#19896=CARTESIAN_POINT('Origin',(0.,-2.05,0.)) ;
#19897=CARTESIAN_POINT('',(-12.5,-0.0999999999999999,1.53080849893419E-15)) ;
#19898=CARTESIAN_POINT('Origin',(0.,-0.0999999999999999,0.)) ;
#19899=CARTESIAN_POINT('',(-12.5,-4.,1.53080849893419E-15)) ;
#19900=CARTESIAN_POINT('',(-12.5,-2.05,1.53080849893419E-15)) ;
#19901=CARTESIAN_POINT('Origin',(0.,-4.,0.)) ;
#19902=CARTESIAN_POINT('',(8.97223799923196,-4.,-8.70338700076804)) ;
#19903=CARTESIAN_POINT('Origin',(0.,-4.,0.)) ;
#19904=CARTESIAN_POINT('',(8.97223799923192,-3.6,-8.70338700076808)) ;
#19905=CARTESIAN_POINT('',(8.97223799923192,-4.7,-8.70338700076808)) ;
#19906=CARTESIAN_POINT('',(8.70338700076808,-3.6,-8.97223799923192)) ;
#19907=CARTESIAN_POINT('Origin',(0.,-3.6,0.)) ;
#19908=CARTESIAN_POINT('',(8.70338700076804,-4.,-8.97223799923196)) ;
#19909=CARTESIAN_POINT('',(8.70338700076808,-4.7,-8.97223799923192)) ;
#19910=CARTESIAN_POINT('Origin',(0.,-4.,0.)) ;
#19911=CARTESIAN_POINT('',(-1.5,-1.8,-12.4096736459909)) ;
#19912=CARTESIAN_POINT('',(-4.5,-1.8,-11.6619037896906)) ;
#19913=CARTESIAN_POINT('Ctrl Pts',(-1.5,-1.8,-12.4096736459909)) ;
#19914=CARTESIAN_POINT('Ctrl Pts',(-1.5,-1.61196600654566,-12.4096736459909)) ;
#19915=CARTESIAN_POINT('Ctrl Pts',(-1.53753764650229,-1.41147435037358,
-12.4053162844128)) ;
#19916=CARTESIAN_POINT('Ctrl Pts',(-1.6517341137174,-1.13508183989584,-12.3904498694233)) ;
#19917=CARTESIAN_POINT('Ctrl Pts',(-1.69911200155108,-1.04678132995196,
-12.3841054114811)) ;
#19918=CARTESIAN_POINT('Ctrl Pts',(-1.80844505033484,-0.883569560086197,
-12.3686124903528)) ;
#19919=CARTESIAN_POINT('Ctrl Pts',(-1.87040554697203,-0.808663104083316,
-12.3594510770994)) ;
#19920=CARTESIAN_POINT('Ctrl Pts',(-2.00366337658874,-0.674636282719867,
-12.3385567824571)) ;
#19921=CARTESIAN_POINT('Ctrl Pts',(-2.07973539361739,-0.611285895478787,
-12.3260595439938)) ;
#19922=CARTESIAN_POINT('Ctrl Pts',(-2.24505223667302,-0.500006906723129,
-12.2970233651971)) ;
#19923=CARTESIAN_POINT('Ctrl Pts',(-2.33429019684881,-0.452070861236452,
-12.2804738646022)) ;
#19924=CARTESIAN_POINT('Ctrl Pts',(-2.51988844594125,-0.375368333774488,
-12.2437376355435)) ;
#19925=CARTESIAN_POINT('Ctrl Pts',(-2.61639808467943,-0.346536928463552,
-12.2235131445539)) ;
#19926=CARTESIAN_POINT('Ctrl Pts',(-2.80979164782945,-0.308850741038295,
-12.1805124452298)) ;
#19927=CARTESIAN_POINT('Ctrl Pts',(-2.90667569879011,-0.3,-12.1577332645547)) ;
#19928=CARTESIAN_POINT('Ctrl Pts',(-3.19117405971703,-0.3,-12.0873979601089)) ;
#19929=CARTESIAN_POINT('Ctrl Pts',(-3.39395738819548,-0.338648265257061,
-12.0319909475619)) ;
#19930=CARTESIAN_POINT('Ctrl Pts',(-3.76627999316394,-0.494792641049793,
-11.9206915878575)) ;
#19931=CARTESIAN_POINT('Ctrl Pts',(-3.93590065069828,-0.61225551516906,
-11.8650249831913)) ;
#19932=CARTESIAN_POINT('Ctrl Pts',(-4.19851097400854,-0.879581031518828,
-11.7745897312595)) ;
#19933=CARTESIAN_POINT('Ctrl Pts',(-4.31145091679816,-1.04551443822509,
-11.7331953681633)) ;
#19934=CARTESIAN_POINT('Ctrl Pts',(-4.42454131034426,-1.31992710340207,
-11.6908107024705)) ;
#19935=CARTESIAN_POINT('Ctrl Pts',(-4.45323046108314,-1.41557935260616,
-11.6798607302848)) ;
#19936=CARTESIAN_POINT('Ctrl Pts',(-4.49096465856084,-1.60847351660445,
-11.6654037501561)) ;
#19937=CARTESIAN_POINT('Ctrl Pts',(-4.5,-1.70571785795988,-11.6619037896906)) ;
#19938=CARTESIAN_POINT('Ctrl Pts',(-4.5,-1.8,-11.6619037896906)) ;
#19939=CARTESIAN_POINT('Ctrl Pts',(-4.5,-1.8,-11.6619037896906)) ;
#19940=CARTESIAN_POINT('Ctrl Pts',(-4.5,-1.89428214204012,-11.6619037896906)) ;
#19941=CARTESIAN_POINT('Ctrl Pts',(-4.49096465856084,-1.99152648339555,
-11.6654037501561)) ;
#19942=CARTESIAN_POINT('Ctrl Pts',(-4.45323046108314,-2.18442064739384,
-11.6798607302848)) ;
#19943=CARTESIAN_POINT('Ctrl Pts',(-4.42454131034426,-2.28007289659793,
-11.6908107024705)) ;
#19944=CARTESIAN_POINT('Ctrl Pts',(-4.31145091679816,-2.55448556177491,
-11.7331953681633)) ;
#19945=CARTESIAN_POINT('Ctrl Pts',(-4.19851097400854,-2.72041896848117,
-11.7745897312595)) ;
#19946=CARTESIAN_POINT('Ctrl Pts',(-3.93590065069828,-2.98774448483094,
-11.8650249831913)) ;
#19947=CARTESIAN_POINT('Ctrl Pts',(-3.76627999316394,-3.10520735895021,
-11.9206915878575)) ;
#19948=CARTESIAN_POINT('Ctrl Pts',(-3.39395738819548,-3.26135173474294,
-12.0319909475619)) ;
#19949=CARTESIAN_POINT('Ctrl Pts',(-3.19117405971703,-3.3,-12.0873979601089)) ;
#19950=CARTESIAN_POINT('Ctrl Pts',(-2.90667569879011,-3.3,-12.1577332645547)) ;
#19951=CARTESIAN_POINT('Ctrl Pts',(-2.80979164782945,-3.29114925896171,
-12.1805124452298)) ;
#19952=CARTESIAN_POINT('Ctrl Pts',(-2.61639808467943,-3.25346307153645,
-12.2235131445539)) ;
#19953=CARTESIAN_POINT('Ctrl Pts',(-2.51988844594125,-3.22463166622551,
-12.2437376355435)) ;
#19954=CARTESIAN_POINT('Ctrl Pts',(-2.33429019684881,-3.14792913876355,
-12.2804738646022)) ;
#19955=CARTESIAN_POINT('Ctrl Pts',(-2.24505223667302,-3.09999309327687,
-12.2970233651971)) ;
#19956=CARTESIAN_POINT('Ctrl Pts',(-2.07973539361739,-2.98871410452121,
-12.3260595439938)) ;
#19957=CARTESIAN_POINT('Ctrl Pts',(-2.00366337658874,-2.92536371728013,
-12.3385567824571)) ;
#19958=CARTESIAN_POINT('Ctrl Pts',(-1.87040554697204,-2.79133689591668,
-12.3594510770994)) ;
#19959=CARTESIAN_POINT('Ctrl Pts',(-1.80844505033484,-2.7164304399138,-12.3686124903528)) ;
#19960=CARTESIAN_POINT('Ctrl Pts',(-1.69911200155108,-2.55321867004804,
-12.3841054114811)) ;
#19961=CARTESIAN_POINT('Ctrl Pts',(-1.6517341137174,-2.46491816010416,-12.3904498694233)) ;
#19962=CARTESIAN_POINT('Ctrl Pts',(-1.53753764650229,-2.18852564962642,
-12.4053162844128)) ;
#19963=CARTESIAN_POINT('Ctrl Pts',(-1.5,-1.98803399345434,-12.4096736459909)) ;
#19964=CARTESIAN_POINT('Ctrl Pts',(-1.5,-1.8,-12.4096736459909)) ;
#19965=CARTESIAN_POINT('Origin',(-3.,-1.8,-11.5)) ;
#19966=CARTESIAN_POINT('',(-4.1,-1.8,-13.)) ;
#19967=CARTESIAN_POINT('Origin',(-3.,-1.8,-13.)) ;
#19968=CARTESIAN_POINT('',(-4.1,-1.8,-11.5)) ;
#19969=CARTESIAN_POINT('Origin',(-3.,-1.8,-11.2)) ;
#19970=CARTESIAN_POINT('Origin',(-3.,-1.8,-12.1)) ;
#19971=CARTESIAN_POINT('',(-4.5,-1.8,-13.)) ;
#19972=CARTESIAN_POINT('',(-4.5,-1.8,-12.1)) ;
#19973=CARTESIAN_POINT('Origin',(-3.,-1.8,-13.)) ;
#19974=CARTESIAN_POINT('Origin',(-3.,-1.8,-12.1)) ;
#19975=CARTESIAN_POINT('Origin',(-3.,-1.8,-11.2)) ;
#19976=CARTESIAN_POINT('Origin',(-3.,-1.8,-13.)) ;
#19977=CARTESIAN_POINT('Origin',(-3.,-1.8,-11.2)) ;
#19978=CARTESIAN_POINT('Origin',(8.,-3.,-8.)) ;
#19979=CARTESIAN_POINT('Origin',(8.,-3.,-8.)) ;
#19980=CARTESIAN_POINT('Origin',(8.,-4.65,-8.)) ;
#19981=CARTESIAN_POINT('',(7.1,-5.8,-8.)) ;
#19982=CARTESIAN_POINT('Origin',(8.,-5.8,-8.)) ;
#19983=CARTESIAN_POINT('',(7.1,-4.65,-8.)) ;
#19984=CARTESIAN_POINT('Origin',(8.,-3.6,-8.)) ;
#19985=CARTESIAN_POINT('Origin',(8.,-3.6,-8.)) ;
#19986=CARTESIAN_POINT('Origin',(8.,-4.7,-8.)) ;
#19987=CARTESIAN_POINT('',(6.8,-4.,-8.)) ;
#19988=CARTESIAN_POINT('Origin',(8.,-4.,-8.)) ;
#19989=CARTESIAN_POINT('',(6.8,-5.8,-8.)) ;
#19990=CARTESIAN_POINT('',(6.8,-4.7,-8.)) ;
#19991=CARTESIAN_POINT('Origin',(8.,-5.8,-8.)) ;
#19992=CARTESIAN_POINT('Origin',(8.,-4.,-8.)) ;
#19993=CARTESIAN_POINT('Origin',(8.,-5.8,-8.)) ;
#19994=CARTESIAN_POINT('Origin',(0.,-4.,0.)) ;
#19995=CARTESIAN_POINT('',(-2.5,-4.,3.06161699786838E-16)) ;
#19996=CARTESIAN_POINT('Origin',(0.,-4.,0.)) ;
#19997=CARTESIAN_POINT('Origin',(0.,-3.8,0.)) ;
#19998=CARTESIAN_POINT('',(-1.5,-4.,1.83697019872103E-16)) ;
#19999=CARTESIAN_POINT('Origin',(0.,-4.,0.)) ;
#20000=CARTESIAN_POINT('',(-1.5,-3.6,-1.83697019872103E-16)) ;
#20001=CARTESIAN_POINT('',(-1.5,-3.8,1.83697019872103E-16)) ;
#20002=CARTESIAN_POINT('Origin',(0.,-3.6,0.)) ;
#20003=CARTESIAN_POINT('Origin',(0.,-2.95,0.)) ;
#20004=CARTESIAN_POINT('',(-1.75,-3.6,2.14313189850787E-16)) ;
#20005=CARTESIAN_POINT('Origin',(0.,-3.6,0.)) ;
#20006=CARTESIAN_POINT('',(-1.75,-2.4,-2.14313189850787E-16)) ;
#20007=CARTESIAN_POINT('',(-1.75,-2.95,2.14313189850787E-16)) ;
#20008=CARTESIAN_POINT('Origin',(0.,-2.4,0.)) ;
#20009=CARTESIAN_POINT('Origin',(0.,-3.6,0.)) ;
#20010=CARTESIAN_POINT('Origin',(0.,-4.85,0.)) ;
#20011=CARTESIAN_POINT('',(-1.75,-5.6,2.14313189850787E-16)) ;
#20012=CARTESIAN_POINT('Origin',(0.,-5.6,0.)) ;
#20013=CARTESIAN_POINT('',(-1.75,-4.,2.14313189850787E-16)) ;
#20014=CARTESIAN_POINT('',(-1.75,-4.85,2.14313189850787E-16)) ;
#20015=CARTESIAN_POINT('Origin',(0.,-4.,0.)) ;
#20016=CARTESIAN_POINT('Origin',(0.,-4.,0.)) ;
#20017=CARTESIAN_POINT('Origin',(0.,-3.,0.)) ;
#20018=CARTESIAN_POINT('',(-2.5,-2.4,3.06161699786838E-16)) ;
#20019=CARTESIAN_POINT('Origin',(0.,-2.4,0.)) ;
#20020=CARTESIAN_POINT('',(-2.5,-3.,3.06161699786838E-16)) ;
#20021=CARTESIAN_POINT('Origin',(0.,-2.4,0.)) ;
#20022=CARTESIAN_POINT('Origin',(0.,-4.6,0.)) ;
#20023=CARTESIAN_POINT('',(-2.5,-5.6,3.06161699786838E-16)) ;
#20024=CARTESIAN_POINT('',(-2.5,-4.6,3.06161699786838E-16)) ;
#20025=CARTESIAN_POINT('Origin',(0.,-5.6,0.)) ;
#20026=CARTESIAN_POINT('Origin',(0.,-5.6,0.)) ;
#20027=CARTESIAN_POINT('Origin',(0.,-0.0999999999999999,0.)) ;
#24535=UNCERTAINTY_MEASURE_WITH_UNIT(LENGTH_MEASURE(0.001),#24629,
'DISTANCE_ACCURACY_VALUE',
'Maximum model space distance between geometric entities at asserted c
onnectivities') ;
#24580=UNCERTAINTY_MEASURE_WITH_UNIT(LENGTH_MEASURE(0.001),#24629,
'DISTANCE_ACCURACY_VALUE',
'Maximum model space distance between geometric entities at asserted c
onnectivities') ;
#24583=(
GEOMETRIC_REPRESENTATION_CONTEXT(3)
GLOBAL_UNCERTAINTY_ASSIGNED_CONTEXT((#24535))
GLOBAL_UNIT_ASSIGNED_CONTEXT((#24629,#24631,#24632))
REPRESENTATION_CONTEXT('','3D')
) ;
#24628=(
GEOMETRIC_REPRESENTATION_CONTEXT(3)
GLOBAL_UNCERTAINTY_ASSIGNED_CONTEXT((#24580))
GLOBAL_UNIT_ASSIGNED_CONTEXT((#24629,#24631,#24632))
REPRESENTATION_CONTEXT('','3D')
) ;
#24629=(
LENGTH_UNIT()
NAMED_UNIT(*)
SI_UNIT(.CENTI.,.METRE.)
) ;
#24631=(
NAMED_UNIT(*)
PLANE_ANGLE_UNIT()
SI_UNIT($,.RADIAN.)
) ;
#24632=(
NAMED_UNIT(*)
SI_UNIT($,.STERADIAN.)
SOLID_ANGLE_UNIT()
) ;
#24635=SHAPE_DEFINITION_REPRESENTATION(#24682,#24793) ;
#24682=PRODUCT_DEFINITION_SHAPE('',$,#24841) ;
#24793=SHAPE_REPRESENTATION('',(#13654),#24583) ;
#24838=PRODUCT_DEFINITION_CONTEXT('part definition',#24981,'design') ;
#24841=PRODUCT_DEFINITION('REAR_SHELL_ENCLOSURE',
'REAR_SHELL_ENCLOSURE',#24888,#24838) ;
#24888=PRODUCT_DEFINITION_FORMATION('',$,#24985) ;
#24981=APPLICATION_CONTEXT(
'Core Data for Automotive Mechanical Design Process') ;
#24982=PRODUCT_CONTEXT('part definition',#24981,'mechanical') ;
#24985=PRODUCT('REAR_SHELL_ENCLOSURE','REAR_SHELL_ENCLOSURE',$,(#24982)) ;
#25031=PRESENTATION_STYLE_ASSIGNMENT((#25041)) ;
#25041=SURFACE_STYLE_USAGE(.BOTH.,#25051) ;
#25051=SURFACE_SIDE_STYLE('',(#25061)) ;
#25061=SURFACE_STYLE_FILL_AREA(#25071) ;
#25071=FILL_AREA_STYLE('Aluminum - Satin',(#25081)) ;
#25081=FILL_AREA_STYLE_COLOUR('Aluminum - Satin',#25091) ;
#25091=COLOUR_RGB('Aluminum - Satin', 0.40784314, 0.44705882, 0.49803922) ;
ENDSEC;
END-ISO-10303-21;
